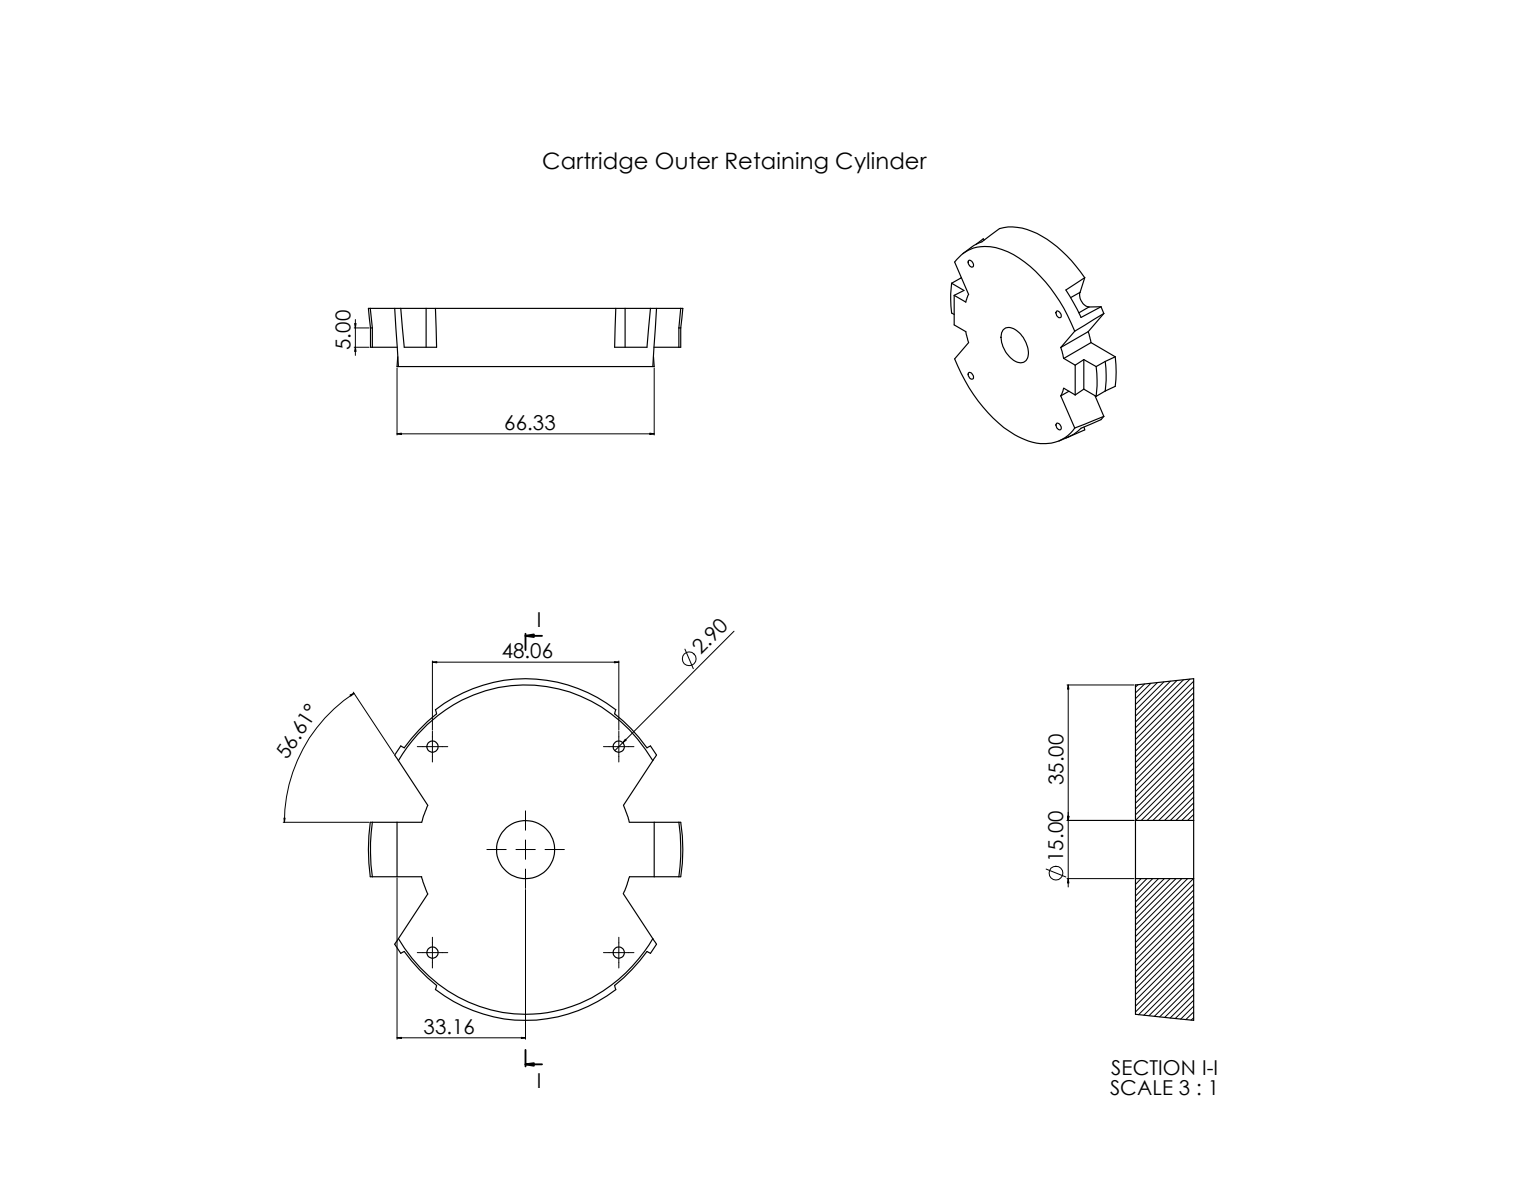
ISO-10303-21;
HEADER;
FILE_DESCRIPTION (('STEP AP214'),
    '1' );
FILE_NAME ('Cartridge Outer Retaining Cylinder.step',
    '2026-10-18T20:16:25',
    ( '' ),
    ( '' ),
    'SwSTEP 2.0',
    'SolidWorks 2025',
    '' );
FILE_SCHEMA (( 'AUTOMOTIVE_DESIGN' ));
ENDSEC;

DATA;
#17=CARTESIAN_POINT ( 'NONE',  ( -9.060903275275968838, 42.96476308719554993, -16.50000000000000000 ) ) ;
#22=EDGE_CURVE ( 'NONE', #25287, #29372, #18804, .T. ) ;
#32=CARTESIAN_POINT ( 'NONE',  ( -20.65888525914364493, -38.75220717792906555, -19.50000000000000355 ) ) ;
#41=CARTESIAN_POINT ( 'NONE',  ( 39.83602371821015709, 11.57901747687536265, -19.50000000000000355 ) ) ;
#46=CARTESIAN_POINT ( 'NONE',  ( -24.03057240117690441, -26.57182937991348481, 26.54355021145563143 ) ) ;
#74=AXIS2_PLACEMENT_3D ( 'NONE', #21270, #28002, #15999 ) ;
#78=DIRECTION ( 'NONE',  ( -1.000000000000000000, 0.000000000000000000, 0.000000000000000000 ) ) ;
#85=CARTESIAN_POINT ( 'NONE',  ( -37.98493438988125348, -11.12428508575252728, -1.500000000000000000 ) ) ;
#92=EDGE_CURVE ( 'NONE', #21118, #30725, #17328, .T. ) ;
#102=CARTESIAN_POINT ( 'NONE',  ( 22.58267429318970443, -26.57182937991349903, 26.54355021145563143 ) ) ;
#111=ORIENTED_EDGE ( 'NONE', *, *, #4642, .T. ) ;
#123=ORIENTED_EDGE ( 'NONE', *, *, #26128, .F. ) ;
#145=LINE ( 'NONE', #9510, #21267 ) ;
#162=AXIS2_PLACEMENT_3D ( 'NONE', #23397, #25742, #23542 ) ;
#169=CARTESIAN_POINT ( 'NONE',  ( 32.24119435725080507, -26.76047165977712794, -16.50000600000000262 ) ) ;
#175=CARTESIAN_POINT ( 'NONE',  ( -10.64374042650075403, -42.96126232887726815, -19.50000000000000355 ) ) ;
#176=CARTESIAN_POINT ( 'NONE',  ( 39.70095622563236049, 7.028748154183632302, -13.16666434799647689 ) ) ;
#184=CARTESIAN_POINT ( 'NONE',  ( -35.76344986165604212, -22.29344514668547461, -19.50000000000000355 ) ) ;
#187=EDGE_CURVE ( 'NONE', #14088, #4162, #7585, .T. ) ;
#226=CARTESIAN_POINT ( 'NONE',  ( 4.770489558936219510E-15, -42.50000000000000000, -1.500000000000000000 ) ) ;
#229=DIRECTION ( 'NONE',  ( -0.000000000000000000, -0.000000000000000000, -1.000000000000000000 ) ) ;
#231=CARTESIAN_POINT ( 'NONE',  ( 32.74775157611827581, 27.21557300921217859, -19.50000000000000355 ) ) ;
#253=CARTESIAN_POINT ( 'NONE',  ( 11.29353189506152511, 42.33618545487009754, -16.50000000000000355 ) ) ;
#258=PLANE ( 'NONE',  #5321 ) ;
#261=PLANE ( 'NONE',  #7575 ) ;
#285=CARTESIAN_POINT ( 'NONE',  ( 31.61046531718064045, -26.43913157134468861, -9.833326303308560057 ) ) ;
#301=CARTESIAN_POINT ( 'NONE',  ( 39.52380524535330153, 7.028748154198969367, -6.500000000000000888 ) ) ;
#313=AXIS2_PLACEMENT_3D ( 'NONE', #7814, #17164, #27009 ) ;
#326=VECTOR ( 'NONE', #28352, 1000.000000000000000 ) ;
#331=AXIS2_PLACEMENT_3D ( 'NONE', #19612, #5728, #15222 ) ;
#333=CARTESIAN_POINT ( 'NONE',  ( -39.00000000000000000, 5.563236990218665134, -1.500000000000000000 ) ) ;
#334=DIRECTION ( 'NONE',  ( 1.000000000000000000, 0.000000000000000000, 0.000000000000000000 ) ) ;
#335=ORIENTED_EDGE ( 'NONE', *, *, #27473, .T. ) ;
#342=CARTESIAN_POINT ( 'NONE',  ( -19.64114023396061981, 37.13592150528867109, -1.500000000000000000 ) ) ;
#347=CARTESIAN_POINT ( 'NONE',  ( 33.67904611720809527, -24.24635140547922418, -14.83330431372250935 ) ) ;
#349=AXIS2_PLACEMENT_3D ( 'NONE', #29658, #10628, #8296 ) ;
#401=CARTESIAN_POINT ( 'NONE',  ( -33.78553954455730235, -24.40792764007751359, -16.50000000000000000 ) ) ;
#407=LINE ( 'NONE', #9924, #2084 ) ;
#434=EDGE_LOOP ( 'NONE', ( #12928, #30003 ) ) ;
#443=DIRECTION ( 'NONE',  ( -0.000000000000000000, -0.000000000000000000, 1.000000000000000000 ) ) ;
#448=ORIENTED_EDGE ( 'NONE', *, *, #24131, .T. ) ;
#455=EDGE_CURVE ( 'NONE', #752, #3032, #6774, .T. ) ;
#471=DIRECTION ( 'NONE',  ( -0.8910248307962437275, 0.4539545692076742966, 0.000000000000000000 ) ) ;
#477=VERTEX_POINT ( 'NONE', #3410 ) ;
#484=LINE ( 'NONE', #7511, #24812 ) ;
#496=CARTESIAN_POINT ( 'NONE',  ( -10.64374042650306862, 42.96126232887723972, -19.50000000000000355 ) ) ;
#503=CARTESIAN_POINT ( 'NONE',  ( -5.105024945673440229, 42.22604126506271172, -1.500000000000000000 ) ) ;
#510=CARTESIAN_POINT ( 'NONE',  ( -33.78553954455730235, -24.40792764007751359, -16.50000000000000000 ) ) ;
#522=CARTESIAN_POINT ( 'NONE',  ( -24.03057240117690441, -26.57182937991348481, -6.499999999999999112 ) ) ;
#534=ORIENTED_EDGE ( 'NONE', *, *, #649, .F. ) ;
#544=VERTEX_POINT ( 'NONE', #30627 ) ;
#546=CARTESIAN_POINT ( 'NONE',  ( -33.57242512144540569, -24.08458161880429316, -13.16663720046962816 ) ) ;
#559=FACE_BOUND ( 'NONE', #17141, .T. ) ;
#571=CARTESIAN_POINT ( 'NONE',  ( 25.47847050916411504, 26.57182937991349903, -6.499999999999999112 ) ) ;
#601=ORIENTED_EDGE ( 'NONE', *, *, #19478, .T. ) ;
#626=ADVANCED_FACE ( 'NONE', ( #10658 ), #17680, .F. ) ;
#645=CARTESIAN_POINT ( 'NONE',  ( -26.80246859415415273, 7.028748154183637631, -1.499999999999999556 ) ) ;
#649=EDGE_CURVE ( 'NONE', #21864, #12141, #26737, .T. ) ;
#653=CARTESIAN_POINT ( 'NONE',  ( -39.00000000000000000, 5.563236990218665134, -1.500000000000000000 ) ) ;
#709=ORIENTED_EDGE ( 'NONE', *, *, #2670, .T. ) ;
#721=ADVANCED_FACE ( 'NONE', ( #3498 ), #3184, .T. ) ;
#730=PLANE ( 'NONE',  #331 ) ;
#732=CARTESIAN_POINT ( 'NONE',  ( 40.35867887216814864, 4.697862823546318012, -16.50000000000000000 ) ) ;
#752=VERTEX_POINT ( 'NONE', #835 ) ;
#762=CARTESIAN_POINT ( 'NONE',  ( -31.45274955327688460, -26.35877938677512233, -8.166661938620272565 ) ) ;
#769=ORIENTED_EDGE ( 'NONE', *, *, #21940, .F. ) ;
#792=CARTESIAN_POINT ( 'NONE',  ( 4.336808689942017736E-16, 42.50000000000000000, -1.500000000000000000 ) ) ;
#797=CARTESIAN_POINT ( 'NONE',  ( 0.000000000000000000, 0.000000000000000000, -1.500000000000000000 ) ) ;
#802=CARTESIAN_POINT ( 'NONE',  ( 10.11202017158399968, 41.14070756921128691, -1.500000000000000000 ) ) ;
#812=CARTESIAN_POINT ( 'NONE',  ( 32.82330813384209023, -22.94799032726822929, -1.500000000000000000 ) ) ;
#814=CARTESIAN_POINT ( 'NONE',  ( 32.51029041841470502, 26.37763988598561937, -16.50000000000000000 ) ) ;
#828=CARTESIAN_POINT ( 'NONE',  ( -20.71335220384823117, 27.86167394782616213, -16.50000600000000262 ) ) ;
#835=CARTESIAN_POINT ( 'NONE',  ( -33.16313691975489064, 7.028748154183637631, -1.500000000000000000 ) ) ;
#844=CARTESIAN_POINT ( 'NONE',  ( 5.105024945674004222, 42.22604126506330857, -1.500000000000000000 ) ) ;
#898=EDGE_LOOP ( 'NONE', ( #12196, #14932, #9204, #16861 ) ) ;
#911=CARTESIAN_POINT ( 'NONE',  ( 31.45274955338841494, -26.35877938683194088, -8.166661939779828572 ) ) ;
#924=AXIS2_PLACEMENT_3D ( 'NONE', #17670, #19692, #8017 ) ;
#981=DIRECTION ( 'NONE',  ( -0.8910248307962436165, -0.4539545692076747407, -0.000000000000000000 ) ) ;
#1013=CARTESIAN_POINT ( 'NONE',  ( -39.83602371821029919, -11.57901747687044924, -19.50000000000000355 ) ) ;
#1051=FACE_OUTER_BOUND ( 'NONE', #29406, .T. ) ;
#1052=EDGE_CURVE ( 'NONE', #4045, #16098, #4383, .T. ) ;
#1095=B_SPLINE_CURVE_WITH_KNOTS ( 'NONE', 3,
 ( #4359, #13883, #26037, #23676 ),
 .UNSPECIFIED., .F., .F.,
 ( 4, 4 ),
 ( 0.000000000000000000, 0.1536962897835600916 ),
 .UNSPECIFIED. ) ;
#1111=CARTESIAN_POINT ( 'NONE',  ( 29.15452456067735199, 29.11038375076175555, -6.500000000000000888 ) ) ;
#1115=CARTESIAN_POINT ( 'NONE',  ( -19.64114023396061981, 37.13592150528867109, -1.500000000000000000 ) ) ;
#1116=FACE_OUTER_BOUND ( 'NONE', #26170, .T. ) ;
#1153=EDGE_CURVE ( 'NONE', #11716, #4151, #9442, .T. ) ;
#1156=CARTESIAN_POINT ( 'NONE',  ( -35.76344986165608475, 22.29344514668535027, -19.50000000000000355 ) ) ;
#1162=CARTESIAN_POINT ( 'NONE',  ( 10.11202017158399968, 41.14070756921128691, -1.500000000000000000 ) ) ;
#1170=CARTESIAN_POINT ( 'NONE',  ( 5.374868878255610660, 44.10336124695606230, -19.50000000000000355 ) ) ;
#1181=DIRECTION ( 'NONE',  ( 0.000000000000000000, 0.000000000000000000, -1.000000000000000000 ) ) ;
#1199=EDGE_CURVE ( 'NONE', #24108, #2130, #15785, .T. ) ;
#1208=CARTESIAN_POINT ( 'NONE',  ( 25.19442432473618254, -35.44676296258426618, -19.50000000000000355 ) ) ;
#1246=ORIENTED_EDGE ( 'NONE', *, *, #13192, .F. ) ;
#1260=LINE ( 'NONE', #29338, #27317 ) ;
#1282=LINE ( 'NONE', #15460, #19231 ) ;
#1300=CARTESIAN_POINT ( 'NONE',  ( -24.98398214727286515, 23.12412086524405908, -16.50001200000000523 ) ) ;
#1302=CARTESIAN_POINT ( 'NONE',  ( -12.33859880789482233, 8.132258305203423632, -1.500000000000000000 ) ) ;
#1308=AXIS2_PLACEMENT_3D ( 'NONE', #17106, #19296, #2769 ) ;
#1310=CARTESIAN_POINT ( 'NONE',  ( -35.78163722268750746, -27.43648963448195133, -11.49999999999999645 ) ) ;
#1311=CARTESIAN_POINT ( 'NONE',  ( 35.76344986163714168, -22.29344514668044752, -19.50000000000000355 ) ) ;
#1317=CARTESIAN_POINT ( 'NONE',  ( -5.105024945675580739, -42.22604126506273303, -1.500000000000000000 ) ) ;
#1322=FACE_OUTER_BOUND ( 'NONE', #29141, .T. ) ;
#1332=CARTESIAN_POINT ( 'NONE',  ( 26.80246859415415273, -7.028748154183637631, -16.50000000000000000 ) ) ;
#1335=PLANE ( 'NONE',  #29203 ) ;
#1357=CARTESIAN_POINT ( 'NONE',  ( -40.89187623478217404, 5.790488632116478129, -19.50000000000000355 ) ) ;
#1362=CARTESIAN_POINT ( 'NONE',  ( 23.27838111857050407, -36.10018641471199174, -16.50000599999999906 ) ) ;
#1378=CARTESIAN_POINT ( 'NONE',  ( 24.03057240117691862, -26.57182937991349903, -6.500000000000000888 ) ) ;
#1393=ORIENTED_EDGE ( 'NONE', *, *, #9979, .F. ) ;
#1401=ORIENTED_EDGE ( 'NONE', *, *, #20994, .F. ) ;
#1408=CIRCLE ( 'NONE', #17835, 27.70876437800068359 ) ;
#1421=ADVANCED_FACE ( 'NONE', ( #4031 ), #18074, .F. ) ;
#1434=CARTESIAN_POINT ( 'NONE',  ( -26.80246859415415273, 7.028748154183637631, -16.50000000000000000 ) ) ;
#1466=CARTESIAN_POINT ( 'NONE',  ( -22.85987860430571317, -23.19171692911513460, -16.50001200000000168 ) ) ;
#1475=LINE ( 'NONE', #15646, #18551 ) ;
#1477=CARTESIAN_POINT ( 'NONE',  ( 2.687479362164894248, -44.39187623478217404, -19.50000000000000355 ) ) ;
#1482=CARTESIAN_POINT ( 'NONE',  ( -39.83602371821034183, 11.57901747687032490, -19.50000000000000355 ) ) ;
#1484=CARTESIAN_POINT ( 'NONE',  ( 24.03057240117691862, 26.57182937991349903, -6.499999999999999112 ) ) ;
#1488=CARTESIAN_POINT ( 'NONE',  ( 39.00000000000000000, -5.563236990218592304, -1.500000000000000000 ) ) ;
#1512=DIRECTION ( 'NONE',  ( 0.5503133621338236470, -0.8349582046168341209, -0.000000000000000000 ) ) ;
#1516=CARTESIAN_POINT ( 'NONE',  ( -32.74775157610409337, 27.21557300919391054, -19.50000000000000355 ) ) ;
#1569=EDGE_LOOP ( 'NONE', ( #15158, #10530, #11871, #10690 ) ) ;
#1574=B_SPLINE_CURVE_WITH_KNOTS ( 'NONE', 3,
 ( #9873, #15005, #12688, #10176, #510 ),
 .UNSPECIFIED., .F., .F.,
 ( 4, 1, 4 ),
 ( 0.1429309129599393158, 0.1481973127024909243, 0.1534637124450425050 ),
 .UNSPECIFIED. ) ;
#1602=AXIS2_PLACEMENT_3D ( 'NONE', #1378, #19360, #7512 ) ;
#1605=CARTESIAN_POINT ( 'NONE',  ( 39.87350638640253919, -4.706224724400463799, -6.500000000000000888 ) ) ;
#1621=ORIENTED_EDGE ( 'NONE', *, *, #4317, .F. ) ;
#1629=CARTESIAN_POINT ( 'NONE',  ( -19.64114023396061981, 37.13592150528867109, -1.500000000000000000 ) ) ;
#1630=CARTESIAN_POINT ( 'NONE',  ( -22.94541271838176044, 35.03073867844246081, -6.500000000000000888 ) ) ;
#1639=CARTESIAN_POINT ( 'NONE',  ( -5.374868878256215510, -44.10336124695545124, -19.50000000000000355 ) ) ;
#1654=CARTESIAN_POINT ( 'NONE',  ( 24.73258466867350336, -33.64422401625958514, -6.500000000000000888 ) ) ;
#1655=CARTESIAN_POINT ( 'NONE',  ( 35.78163722268750746, 27.43648963448195133, -11.49999999999999645 ) ) ;
#1667=CARTESIAN_POINT ( 'NONE',  ( 24.03057240117691862, 26.57182937991349903, -6.500000000000000888 ) ) ;
#1750=ADVANCED_FACE ( 'NONE', ( #21628, #14614 ), #24117, .T. ) ;
#1754=CARTESIAN_POINT ( 'NONE',  ( -25.64627119138473432, -23.40052582045089480, -16.50000600000000262 ) ) ;
#1756=ADVANCED_FACE ( 'NONE', ( #10234 ), #12279, .F. ) ;
#1757=CARTESIAN_POINT ( 'NONE',  ( 24.03057240117690441, -26.57182937991349903, 26.54355021145563143 ) ) ;
#1763=CARTESIAN_POINT ( 'NONE',  ( 0.000000000000000000, 44.39187623478217404, -19.50000000000000355 ) ) ;
#1781=CARTESIAN_POINT ( 'NONE',  ( -2.687479363073305372, 44.39187623477332068, -19.50000000000000355 ) ) ;
#1812=CARTESIAN_POINT ( 'NONE',  ( 33.67904611717059993, 24.24635140542181233, -14.83330431306680453 ) ) ;
#1847=CIRCLE ( 'NONE', #17271, 27.70876437800068359 ) ;
#1863=VERTEX_POINT ( 'NONE', #23003 ) ;
#1864=CARTESIAN_POINT ( 'NONE',  ( -24.73258466867759608, 33.64422401626517001, -6.500000000000000888 ) ) ;
#1869=LINE ( 'NONE', #6846, #8646 ) ;
#1896=EDGE_LOOP ( 'NONE', ( #27103, #9157, #6706, #24049 ) ) ;
#1902=CARTESIAN_POINT ( 'NONE',  ( -20.29038667444665833, 38.16990472509154841, -16.50000000000000000 ) ) ;
#1907=CARTESIAN_POINT ( 'NONE',  ( -24.98398214727285804, -23.12412086524405908, -16.50001200000000523 ) ) ;
#1908=CARTESIAN_POINT ( 'NONE',  ( -25.64627119138473788, 23.40052582045089480, -16.50000000000000000 ) ) ;
#1912=ORIENTED_EDGE ( 'NONE', *, *, #28902, .T. ) ;
#1932=CARTESIAN_POINT ( 'NONE',  ( -23.96732207938974213, -33.98584080153308662, -1.500000000000000000 ) ) ;
#1958=LINE ( 'NONE', #18960, #28468 ) ;
#1961=DIRECTION ( 'NONE',  ( 0.000000000000000000, 1.000000000000000000, -0.000000000000000000 ) ) ;
#1964=CARTESIAN_POINT ( 'NONE',  ( 12.56641067637628240, -40.32935944494942504, -1.500000000000000000 ) ) ;
#1966=CARTESIAN_POINT ( 'NONE',  ( -26.80246859415415273, -7.028748154183645624, -1.499999999999999556 ) ) ;
#1970=CIRCLE ( 'NONE', #4441, 1.447898107987198646 ) ;
#1976=EDGE_CURVE ( 'NONE', #12213, #16156, #16385, .T. ) ;
#1989=CARTESIAN_POINT ( 'NONE',  ( 23.06931171825916493, -36.25841434086032677, -16.50000000000000000 ) ) ;
#2009=B_SPLINE_CURVE_WITH_KNOTS ( 'NONE', 3,
 ( #16990, #26512, #16530, #11702, #7021, #23395, #2033, #28545, #21360, #11557 ),
 .UNSPECIFIED., .F., .F.,
 ( 4, 2, 2, 2, 4 ),
 ( 0.08772604163077325767, 0.09629186329443806258, 0.1119390432090576204, 0.1197626331663674271, 0.1275862231236772337 ),
 .UNSPECIFIED. ) ;
#2012=CARTESIAN_POINT ( 'NONE',  ( -24.03057240117691862, 26.57182937991348481, 26.54355021145563143 ) ) ;
#2016=ORIENTED_EDGE ( 'NONE', *, *, #30517, .T. ) ;
#2033=CARTESIAN_POINT ( 'NONE',  ( -10.11202017158466759, 41.14070756921185534, -1.500000000000009992 ) ) ;
#2047=CARTESIAN_POINT ( 'NONE',  ( -19.05926965620446722, 38.91648619949726395, -16.49999999999999289 ) ) ;
#2050=CARTESIAN_POINT ( 'NONE',  ( -39.52380524535562500, 7.028748154183637631, -11.49999999999999645 ) ) ;
#2075=CARTESIAN_POINT ( 'NONE',  ( -34.07766914599908148, -21.40380666528021081, -1.500000000000000000 ) ) ;
#2076=LINE ( 'NONE', #25500, #21890 ) ;
#2084=VECTOR ( 'NONE', #19436, 1000.000000000000000 ) ;
#2093=PRODUCT_DEFINITION ( 'UNKNOWN', '', #6419, #16060 ) ;
#2099=LINE ( 'NONE', #11622, #24469 ) ;
#2109=CARTESIAN_POINT ( 'NONE',  ( -25.19442432475839055, 35.44676296258369064, -19.50000000000000355 ) ) ;
#2127=AXIS2_PLACEMENT_3D ( 'NONE', #16002, #25522, #22698 ) ;
#2130=VERTEX_POINT ( 'NONE', #14428 ) ;
#2131=CARTESIAN_POINT ( 'NONE',  ( -32.82330813384395185, 22.94799032727105370, -1.500000000000000000 ) ) ;
#2135=CARTESIAN_POINT ( 'NONE',  ( 5.229169525036386545, -43.72378943593913192, -16.49999999999999289 ) ) ;
#2161=CARTESIAN_POINT ( 'NONE',  ( 0.000000000000000000, 0.000000000000000000, -16.50000000000000000 ) ) ;
#2195=CARTESIAN_POINT ( 'NONE',  ( 40.05104235265675783, -2.353288714521556191, -6.500000000000000888 ) ) ;
#2214=CARTESIAN_POINT ( 'NONE',  ( 2.552544031601107211, 42.49999999998228617, -1.500000000000000000 ) ) ;
#2215=FACE_OUTER_BOUND ( 'NONE', #8737, .T. ) ;
#2221=CARTESIAN_POINT ( 'NONE',  ( 35.76344986165623396, 22.29344514668041199, -19.50000000000000355 ) ) ;
#2227=ORIENTED_EDGE ( 'NONE', *, *, #29644, .F. ) ;
#2231=VERTEX_POINT ( 'NONE', #10865 ) ;
#2242=DIRECTION ( 'NONE',  ( 1.000000000000000000, -1.559722691008415723E-11, 0.000000000000000000 ) ) ;
#2254=CARTESIAN_POINT ( 'NONE',  ( 32.82330813384209023, -22.94799032726822929, -1.500000000000000000 ) ) ;
#2258=CARTESIAN_POINT ( 'NONE',  ( 5.105024945674004222, 42.22604126506330857, -1.500000000000000000 ) ) ;
#2259=DIRECTION ( 'NONE',  ( -0.000000000000000000, -0.000000000000000000, -1.000000000000000000 ) ) ;
#2261=VERTEX_POINT ( 'NONE', #13366 ) ;
#2270=CARTESIAN_POINT ( 'NONE',  ( -21.58118279630250314, -37.32782027973600947, -16.50000000000000000 ) ) ;
#2292=VERTEX_POINT ( 'NONE', #26986 ) ;
#2297=( NAMED_UNIT ( * ) PLANE_ANGLE_UNIT ( ) SI_UNIT ( $, .RADIAN. ) );
#2298=VERTEX_POINT ( 'NONE', #18040 ) ;
#2305=CARTESIAN_POINT ( 'NONE',  ( 32.24119409414369386, 26.76047229433004659, -16.50000600000000262 ) ) ;
#2332=CARTESIAN_POINT ( 'NONE',  ( 40.05104235265675783, -2.353288714521559744, -11.49999999999999645 ) ) ;
#2355=CARTESIAN_POINT ( 'NONE',  ( -19.85060193104290960, 38.44128451546529845, -16.49999999999999645 ) ) ;
#2366=FACE_OUTER_BOUND ( 'NONE', #5694, .T. ) ;
#2371=CARTESIAN_POINT ( 'NONE',  ( 23.96732207937828463, 33.98584080152456011, -1.500000000000000000 ) ) ;
#2382=CARTESIAN_POINT ( 'NONE',  ( 13.22505861668094340, 42.10773672057246841, -19.50000000000000355 ) ) ;
#2393=CARTESIAN_POINT ( 'NONE',  ( -5.105024945675580739, -42.22604126506273303, -1.500000000000000000 ) ) ;
#2404=VECTOR ( 'NONE', #10692, 1000.000000000000114 ) ;
#2405=LINE ( 'NONE', #17052, #29792 ) ;
#2425=VERTEX_POINT ( 'NONE', #7566 ) ;
#2428=CARTESIAN_POINT ( 'NONE',  ( -19.64114023396299302, -37.13592150529018454, -1.500000000000000000 ) ) ;
#2440=CARTESIAN_POINT ( 'NONE',  ( -33.35889462893121049, -23.76060431981724363, -9.833271596736169684 ) ) ;
#2442=LINE ( 'NONE', #11963, #7867 ) ;
#2478=CARTESIAN_POINT ( 'NONE',  ( 25.23756106473024019, 11.43858098102958287, -11.49999999999999645 ) ) ;
#2482=DIRECTION ( 'NONE',  ( -0.000000000000000000, -0.000000000000000000, -1.000000000000000000 ) ) ;
#2496=CARTESIAN_POINT ( 'NONE',  ( -40.05520443301966083, -7.028746486913004077, -16.50000000000000000 ) ) ;
#2497=CARTESIAN_POINT ( 'NONE',  ( 20.62927206985200712, -25.36120318786823802, -16.50001200000000523 ) ) ;
#2503=ADVANCED_FACE ( 'NONE', ( #10514 ), #6662, .T. ) ;
#2527=CARTESIAN_POINT ( 'NONE',  ( -24.73258466867722660, -33.64422401626472237, -6.500000000000000888 ) ) ;
#2532=CARTESIAN_POINT ( 'NONE',  ( -2.687479363073305372, 44.39187623477332068, -19.50000000000000355 ) ) ;
#2541=CARTESIAN_POINT ( 'NONE',  ( -39.00000000000000000, -5.563236990218529243, -1.500000000000000000 ) ) ;
#2553=CARTESIAN_POINT ( 'NONE',  ( -24.03057240117691862, -26.57182937991349903, -6.500000000000000888 ) ) ;
#2557=EDGE_LOOP ( 'NONE', ( #20705, #9961, #8594, #30062 ) ) ;
#2580=ORIENTED_EDGE ( 'NONE', *, *, #22101, .T. ) ;
#2594=CARTESIAN_POINT ( 'NONE',  ( -22.43745300381736030, -36.72714324444464040, -16.50000000000000000 ) ) ;
#2599=CARTESIAN_POINT ( 'NONE',  ( 16.14703582738955490, 40.45263314063372206, -16.50000000000000711 ) ) ;
#2645=ORIENTED_EDGE ( 'NONE', *, *, #23070, .F. ) ;
#2654=MANIFOLD_SOLID_BREP ( 'Cut-Extrude13', #3869 ) ;
#2658=EDGE_CURVE ( 'NONE', #16156, #16328, #1282, .T. ) ;
#2670=EDGE_CURVE ( 'NONE', #477, #1863, #17345, .T. ) ;
#2679=CARTESIAN_POINT ( 'NONE',  ( -37.98493438988125348, -11.12428508575252728, -1.500000000000000000 ) ) ;
#2690=CARTESIAN_POINT ( 'NONE',  ( 34.07766914600081520, 21.40380666527109810, -1.500000000000000000 ) ) ;
#2698=CYLINDRICAL_SURFACE ( 'NONE', #27387, 3.559164065751841743 ) ;
#2699=ORIENTED_EDGE ( 'NONE', *, *, #23180, .F. ) ;
#2721=CARTESIAN_POINT ( 'NONE',  ( 24.03057240117691862, 26.57182937991349903, -6.500000000000000888 ) ) ;
#2752=ORIENTED_EDGE ( 'NONE', *, *, #25397, .F. ) ;
#2756=CARTESIAN_POINT ( 'NONE',  ( 18.46022885586396356, 39.25482954210340125, -16.49999999999999645 ) ) ;
#2766=DIRECTION ( 'NONE',  ( -0.000000000000000000, -0.000000000000000000, -1.000000000000000000 ) ) ;
#2769=DIRECTION ( 'NONE',  ( -1.000000000000000000, 0.000000000000000000, 0.000000000000000000 ) ) ;
#2815=CARTESIAN_POINT ( 'NONE',  ( 5.204170427930421283E-15, -44.07656352898514740, -16.50000000000000000 ) ) ;
#2823=AXIS2_PLACEMENT_3D ( 'NONE', #19081, #25384, #23019 ) ;
#2824=FACE_OUTER_BOUND ( 'NONE', #13856, .T. ) ;
#2827=CARTESIAN_POINT ( 'NONE',  ( -24.03057240117691862, 26.57182937991348481, -1.500000000000001332 ) ) ;
#2836=CARTESIAN_POINT ( 'NONE',  ( -13.22505861668184046, -42.10773672057003125, -19.50000000000000355 ) ) ;
#2837=CARTESIAN_POINT ( 'NONE',  ( 40.05520497557499482, 7.028746409576331011, -16.50000000000000000 ) ) ;
#2844=CARTESIAN_POINT ( 'NONE',  ( -39.83602371821034183, 11.57901747687032490, -19.50000000000000355 ) ) ;
#2867=CARTESIAN_POINT ( 'NONE',  ( -23.20738078402527549, 23.09073189384302793, -16.50001200000000168 ) ) ;
#2870=CARTESIAN_POINT ( 'NONE',  ( 11.46038621610576236, -42.28394141292588415, -16.50000000000000000 ) ) ;
#2891=EDGE_CURVE ( 'NONE', #25287, #18178, #3562, .T. ) ;
#2900=VECTOR ( 'NONE', #14038, 1000.000000000000114 ) ;
#2902=ORIENTED_EDGE ( 'NONE', *, *, #8502, .F. ) ;
#2912=EDGE_CURVE ( 'NONE', #30328, #18557, #9016, .T. ) ;
#2915=ORIENTED_EDGE ( 'NONE', *, *, #25460, .F. ) ;
#2917=FACE_BOUND ( 'NONE', #16843, .T. ) ;
#2922=DIRECTION ( 'NONE',  ( -1.000000000000000000, 0.000000000000000000, -0.000000000000000000 ) ) ;
#2936=DIRECTION ( 'NONE',  ( -0.000000000000000000, -0.000000000000000000, 1.000000000000000000 ) ) ;
#2995=CARTESIAN_POINT ( 'NONE',  ( 0.000000000000000000, 0.000000000000000000, -1.500000000000001332 ) ) ;
#3001=ORIENTED_EDGE ( 'NONE', *, *, #27898, .T. ) ;
#3006=CARTESIAN_POINT ( 'NONE',  ( 37.98493438989863336, -11.12428508576153341, -1.500000000000000000 ) ) ;
#3007=DIRECTION ( 'NONE',  ( 1.000000000000000000, 0.000000000000000000, 0.000000000000000000 ) ) ;
#3012=ORIENTED_EDGE ( 'NONE', *, *, #18180, .F. ) ;
#3022=CARTESIAN_POINT ( 'NONE',  ( -39.52380524535562500, 7.028748154183637631, -1.499999999999999556 ) ) ;
#3032=VERTEX_POINT ( 'NONE', #16643 ) ;
#3060=CARTESIAN_POINT ( 'NONE',  ( 5.184529477212510784, 43.72990366966700293, -16.50000000000000000 ) ) ;
#3075=ADVANCED_FACE ( 'NONE', ( #21464, #14750, #10079, #559, #2917, #18990 ), #258, .F. ) ;
#3079=DIRECTION ( 'NONE',  ( -1.000000000000000000, 0.000000000000000000, 0.000000000000000000 ) ) ;
#3108=LINE ( 'NONE', #24769, #14010 ) ;
#3125=ORIENTED_EDGE ( 'NONE', *, *, #26838, .F. ) ;
#3129=ORIENTED_EDGE ( 'NONE', *, *, #29186, .T. ) ;
#3148=CARTESIAN_POINT ( 'NONE',  ( -23.96732207939035675, 33.98584080153585774, -1.500000000000000000 ) ) ;
#3156=CARTESIAN_POINT ( 'NONE',  ( -13.22505861668333083, 42.10773672057167261, -19.50000000000000355 ) ) ;
#3165=CARTESIAN_POINT ( 'NONE',  ( 33.25198513809822742, -23.59839681648444554, -8.166573414591441704 ) ) ;
#3176=CARTESIAN_POINT ( 'NONE',  ( 39.52380524535562500, 7.028748154183637631, -6.500000000000000888 ) ) ;
#3184=PLANE ( 'NONE',  #25082 ) ;
#3191=CARTESIAN_POINT ( 'NONE',  ( 2.552544031601107211, 42.49999999998228617, -1.500000000000000000 ) ) ;
#3217=CARTESIAN_POINT ( 'NONE',  ( -26.80246859415415273, 7.028748154183637631, -1.499999999999999556 ) ) ;
#3270=CARTESIAN_POINT ( 'NONE',  ( -20.71335220384823117, 27.86167394782616213, -16.50000600000000262 ) ) ;
#3296=VERTEX_POINT ( 'NONE', #21107 ) ;
#3328=CARTESIAN_POINT ( 'NONE',  ( -22.58267429318971864, 26.57182937991348481, -1.500000000000001332 ) ) ;
#3340=CARTESIAN_POINT ( 'NONE',  ( 31.18700685317242716, 26.11823559933198879, -1.500000000000000000 ) ) ;
#3346=CARTESIAN_POINT ( 'NONE',  ( -31.18700685316100163, -26.11823559932341610, -1.500000000000000000 ) ) ;
#3370=VECTOR ( 'NONE', #14525, 1000.000000000000114 ) ;
#3380=ORIENTED_EDGE ( 'NONE', *, *, #1052, .F. ) ;
#3394=ORIENTED_EDGE ( 'NONE', *, *, #19459, .F. ) ;
#3398=CARTESIAN_POINT ( 'NONE',  ( 40.56744461766400178, 1.008925180279410139, -16.50000000000000000 ) ) ;
#3404=EDGE_LOOP ( 'NONE', ( #25073, #1401, #3581, #18257, #26796, #15185, #9678, #9859, #11224, #26072, #16671, #534, #335, #23589, #5816, #30130, #28609, #20043, #22288, #9616, #21858, #17373, #5302, #7145, #17610, #15610, #17048, #1393, #16611, #14155, #14862, #18230, #16761, #17005, #27766, #9497 ) ) ;
#3410=CARTESIAN_POINT ( 'NONE',  ( -25.64627119138473788, 23.40052582045089480, -16.50000000000000000 ) ) ;
#3447=CARTESIAN_POINT ( 'NONE',  ( -26.80246859415415273, -7.028748154183637631, -1.499999999999999556 ) ) ;
#3498=FACE_OUTER_BOUND ( 'NONE', #18843, .T. ) ;
#3510=ORIENTED_EDGE ( 'NONE', *, *, #19853, .F. ) ;
#3512=CARTESIAN_POINT ( 'NONE',  ( 5.374868878254059013, -44.10336124695543703, -19.50000000000000355 ) ) ;
#3517=AXIS2_PLACEMENT_3D ( 'NONE', #29672, #17356, #13147 ) ;
#3519=CARTESIAN_POINT ( 'NONE',  ( -35.76344986165604212, -22.29344514668547461, -19.50000000000000355 ) ) ;
#3544=CARTESIAN_POINT ( 'NONE',  ( -35.76344986165604212, -22.29344514668547461, -19.50000000000000355 ) ) ;
#3562=LINE ( 'NONE', #7945, #13243 ) ;
#3571=DIRECTION ( 'NONE',  ( -1.000000000000000000, 0.000000000000000000, 0.000000000000000000 ) ) ;
#3580=CARTESIAN_POINT ( 'NONE',  ( -33.16313691975489064, -7.028748154183637631, -1.500000000000000000 ) ) ;
#3581=ORIENTED_EDGE ( 'NONE', *, *, #15915, .F. ) ;
#3604=CARTESIAN_POINT ( 'NONE',  ( 22.94541271837968566, 35.03073867843525591, -6.499999999999999112 ) ) ;
#3637=CARTESIAN_POINT ( 'NONE',  ( -23.22298177193101765, -35.92225147532004570, -14.83329744750909995 ) ) ;
#3659=CARTESIAN_POINT ( 'NONE',  ( 19.64114023396890829, 37.13592150528549496, -1.500000000000000000 ) ) ;
#3660=ADVANCED_FACE ( 'NONE', ( #20244 ), #29771, .T. ) ;
#3662=B_SPLINE_CURVE_WITH_KNOTS ( 'NONE', 3,
 ( #11603, #26682, #7661, #24012, #21523, #19358, #5312, #14520, #13945, #9842 ),
 .UNSPECIFIED., .F., .F.,
 ( 4, 3, 3, 4 ),
 ( -0.005033671592849668641, 0.000000000000000000, 0.005033946531780089662, 0.01006789358107974472 ),
 .UNSPECIFIED. ) ;
#3666=CARTESIAN_POINT ( 'NONE',  ( 12.56641067637329812, 40.32935944495179115, -1.500000000000000000 ) ) ;
#3709=DIRECTION ( 'NONE',  ( -1.000000000000000000, 0.000000000000000000, 0.000000000000000000 ) ) ;
#3721=EDGE_LOOP ( 'NONE', ( #8377, #22423, #28746, #15898 ) ) ;
#3734=PLANE ( 'NONE',  #12264 ) ;
#3753=VERTEX_POINT ( 'NONE', #30223 ) ;
#3795=CARTESIAN_POINT ( 'NONE',  ( -24.03057240117690441, -26.57182937991348481, 26.54355021145563143 ) ) ;
#3797=CARTESIAN_POINT ( 'NONE',  ( -20.71335220384823117, -27.86167394782616213, -16.50000000000000000 ) ) ;
#3806=CARTESIAN_POINT ( 'NONE',  ( -2.687479363073305372, 44.39187623477332068, -19.50000000000000355 ) ) ;
#3811=CARTESIAN_POINT ( 'NONE',  ( 23.96732207937828463, 33.98584080152456011, -1.500000000000000000 ) ) ;
#3817=CARTESIAN_POINT ( 'NONE',  ( 31.18700685317242716, 26.11823559933198879, -1.500000000000000000 ) ) ;
#3829=CARTESIAN_POINT ( 'NONE',  ( 1.734723475976807094E-15, -44.07656352898514740, -6.500000000000000888 ) ) ;
#3859=ORIENTED_EDGE ( 'NONE', *, *, #19661, .T. ) ;
#3861=VECTOR ( 'NONE', #12040, 1000.000000000000000 ) ;
#3869=CLOSED_SHELL ( 'NONE', ( #28448, #2503, #13583, #1756, #8857, #10128, #14330, #27072, #18523, #3075, #9353, #28639, #6406, #4777, #6909, #16272, #15303, #4583, #21564, #15221, #27786, #24242, #626, #1750, #15368, #25391, #20831, #21794, #15982, #23364, #9380, #8644, #8818, #20413, #8615, #9779, #23667, #27306, #5769, #29435, #25776, #12783, #18322, #8982, #7354, #30362, #5241, #3660, #17604, #1421, #24429, #721, #17780, #23893 ) ) ;
#3937=B_SPLINE_SURFACE_WITH_KNOTS ( 'NONE', 3, 1, ( 
 ( #28544, #28395 ),
 ( #30568, #23998 ),
 ( #19177, #2332 ),
 ( #18720, #4678 ),
 ( #28699, #14500 ),
 ( #301, #4827 ) ),
 .UNSPECIFIED., .F., .F., .F.,
 ( 4, 2, 4 ),
 ( 2, 2 ),
 ( 1.408367944307646891, 1.570796326794821507, 1.733224709277728426 ),
 ( 0.000000000000000000, 1.000000000000000000 ),
 .UNSPECIFIED. ) ;
#3940=AXIS2_PLACEMENT_3D ( 'NONE', #5168, #28727, #21687 ) ;
#3952=AXIS2_PLACEMENT_3D ( 'NONE', #11741, #30768, #25935 ) ;
#3969=CARTESIAN_POINT ( 'NONE',  ( 12.56641067637628240, -40.32935944494942504, -1.500000000000000000 ) ) ;
#3973=CARTESIAN_POINT ( 'NONE',  ( -32.74775157610409337, 27.21557300919391054, -19.50000000000000355 ) ) ;
#3979=CARTESIAN_POINT ( 'NONE',  ( 2.687479362164894248, -44.39187623478217404, -19.50000000000000355 ) ) ;
#4002=CARTESIAN_POINT ( 'NONE',  ( -40.05520443301966083, -7.028746486913004077, -16.50000000000000000 ) ) ;
#4025=CARTESIAN_POINT ( 'NONE',  ( 25.47847050916410439, -26.57182937991349903, 26.54355021145563143 ) ) ;
#4031=FACE_OUTER_BOUND ( 'NONE', #21646, .T. ) ;
#4035=ORIENTED_EDGE ( 'NONE', *, *, #10269, .T. ) ;
#4045=VERTEX_POINT ( 'NONE', #29895 ) ;
#4058=EDGE_CURVE ( 'NONE', #6837, #752, #27084, .T. ) ;
#4065=CARTESIAN_POINT ( 'NONE',  ( 31.29501345866090389, 26.27841684422296353, -6.500000000000000888 ) ) ;
#4079=LINE ( 'NONE', #13609, #19373 ) ;
#4084=EDGE_CURVE ( 'NONE', #15207, #7019, #19784, .T. ) ;
#4091=EDGE_LOOP ( 'NONE', ( #13530, #26791, #12899, #4967 ) ) ;
#4096=FACE_OUTER_BOUND ( 'NONE', #11719, .T. ) ;
#4111=CARTESIAN_POINT ( 'NONE',  ( -12.56641067637617759, -40.32935944494947478, -1.500000000000000000 ) ) ;
#4122=CARTESIAN_POINT ( 'NONE',  ( 12.33859880789485253, 8.132258305203430737, -16.50000000000000000 ) ) ;
#4124=CARTESIAN_POINT ( 'NONE',  ( -20.65888525914099105, 38.75220717792564784, -19.50000000000000355 ) ) ;
#4151=VERTEX_POINT ( 'NONE', #6485 ) ;
#4159=CARTESIAN_POINT ( 'NONE',  ( 26.80246859415415273, -7.028748154183637631, -6.500000000000000888 ) ) ;
#4162=VERTEX_POINT ( 'NONE', #18799 ) ;
#4169=CARTESIAN_POINT ( 'NONE',  ( 8.828055718019477638, -43.02192272134110596, -16.50000000000000000 ) ) ;
#4182=VERTEX_POINT ( 'NONE', #4453 ) ;
#4185=EDGE_CURVE ( 'NONE', #15872, #6674, #25382, .T. ) ;
#4208=ORIENTED_EDGE ( 'NONE', *, *, #6336, .T. ) ;
#4218=EDGE_CURVE ( 'NONE', #14001, #13970, #18775, .T. ) ;
#4230=ORIENTED_EDGE ( 'NONE', *, *, #2891, .T. ) ;
#4235=CARTESIAN_POINT ( 'NONE',  ( -20.94685371601454094, 37.75489722317177410, -16.49999999999998934 ) ) ;
#4242=DIRECTION ( 'NONE',  ( -0.000000000000000000, -0.000000000000000000, -1.000000000000000000 ) ) ;
#4250=ORIENTED_EDGE ( 'NONE', *, *, #17204, .F. ) ;
#4254=CARTESIAN_POINT ( 'NONE',  ( -2.552544031601109875, 42.50000000001772094, -1.500000000000000000 ) ) ;
#4264=VERTEX_POINT ( 'NONE', #29080 ) ;
#4269=ORIENTED_EDGE ( 'NONE', *, *, #6714, .T. ) ;
#4279=CARTESIAN_POINT ( 'NONE',  ( -20.71335220384823117, 27.86167394782616213, -16.50000000000000000 ) ) ;
#4296=CARTESIAN_POINT ( 'NONE',  ( -2.687479363073305372, 44.39187623477332068, -19.50000000000000355 ) ) ;
#4298=ORIENTED_EDGE ( 'NONE', *, *, #24131, .F. ) ;
#4307=CARTESIAN_POINT ( 'NONE',  ( -18.92920200386403451, -38.99007567941009711, -16.50000000000000000 ) ) ;
#4311=B_SPLINE_CURVE_WITH_KNOTS ( 'NONE', 3,
 ( #10305, #19822, #5118, #26332, #28979, #5270, #2305 ),
 .UNSPECIFIED., .F., .F.,
 ( 4, 3, 4 ),
 ( 0.000000000000000000, 0.005028111721475434122, 0.01005622344647096392 ),
 .UNSPECIFIED. ) ;
#4317=EDGE_CURVE ( 'NONE', #16098, #16473, #6136, .T. ) ;
#4325=VECTOR ( 'NONE', #2242, 1000.000000000000000 ) ;
#4332=CIRCLE ( 'NONE', #24257, 1.447898107987198646 ) ;
#4337=( NAMED_UNIT ( * ) SI_UNIT ( $, .STERADIAN. ) SOLID_ANGLE_UNIT ( ) );
#4345=LINE ( 'NONE', #11535, #19465 ) ;
#4350=AXIS2_PLACEMENT_3D ( 'NONE', #13291, #27633, #18117 ) ;
#4359=CARTESIAN_POINT ( 'NONE',  ( 20.71335220384823117, -27.86167394782616213, -16.50000600000000262 ) ) ;
#4369=EDGE_LOOP ( 'NONE', ( #25058, #111, #24453, #3394 ) ) ;
#4378=LINE ( 'NONE', #20906, #7453 ) ;
#4383=CIRCLE ( 'NONE', #21814, 7.500000000000000000 ) ;
#4385=CARTESIAN_POINT ( 'NONE',  ( 39.52380524533145945, -7.028748154382047808, -6.500000000000000888 ) ) ;
#4408=CARTESIAN_POINT ( 'NONE',  ( 13.22505861668094340, 42.10773672057246841, -19.50000000000000355 ) ) ;
#4414=CARTESIAN_POINT ( 'NONE',  ( -10.11202017158235833, -41.14070756921188377, -1.500000000000000000 ) ) ;
#4441=AXIS2_PLACEMENT_3D ( 'NONE', #15620, #20461, #29981 ) ;
#4443=ORIENTED_EDGE ( 'NONE', *, *, #19075, .F. ) ;
#4453=CARTESIAN_POINT ( 'NONE',  ( 25.47847050916411504, 26.57182937991349903, -1.500000000000001332 ) ) ;
#4459=PLANE ( 'NONE',  #20543 ) ;
#4463=CARTESIAN_POINT ( 'NONE',  ( 39.00000000000000000, -5.563236990218592304, -1.500000000000000000 ) ) ;
#4469=B_SPLINE_CURVE_WITH_KNOTS ( 'NONE', 1,
 ( #9085, #28113 ),
 .UNSPECIFIED., .F., .F.,
 ( 2, 2 ),
 ( 0.1666666666666667962, 1.000000000000000000 ),
 .UNSPECIFIED. ) ;
#4476=CARTESIAN_POINT ( 'NONE',  ( 24.03057240117690441, -26.57182937991349903, -6.499999999999999112 ) ) ;
#4477=CARTESIAN_POINT ( 'NONE',  ( -16.16747268278624716, -40.42849113817944584, -16.49999999999999645 ) ) ;
#4480=DIRECTION ( 'NONE',  ( -0.000000000000000000, -0.000000000000000000, -1.000000000000000000 ) ) ;
#4486=CARTESIAN_POINT ( 'NONE',  ( 21.14511335159655658, -37.62126931545598296, -16.50000000000000000 ) ) ;
#4489=DIRECTION ( 'NONE',  ( 1.000000000000000000, 0.000000000000000000, 0.000000000000000000 ) ) ;
#4493=ORIENTED_EDGE ( 'NONE', *, *, #2912, .T. ) ;
#4504=PLANE ( 'NONE',  #22888 ) ;
#4542=CARTESIAN_POINT ( 'NONE',  ( -11.30959556923743392, 42.34504995199416300, -16.50000000000000000 ) ) ;
#4556=CARTESIAN_POINT ( 'NONE',  ( 20.65888525914559892, 38.75220717792412728, -19.50000000000000355 ) ) ;
#4557=DIRECTION ( 'NONE',  ( -1.000000000000000000, 0.000000000000000000, 0.000000000000000000 ) ) ;
#4575=CARTESIAN_POINT ( 'NONE',  ( -19.64114023396299302, -37.13592150529018454, -1.500000000000000000 ) ) ;
#4583=ADVANCED_FACE ( 'NONE', ( #2215 ), #26228, .T. ) ;
#4586=DIRECTION ( 'NONE',  ( 0.5503133621338236470, 0.8349582046168341209, 0.000000000000000000 ) ) ;
#4589=DIRECTION ( 'NONE',  ( -0.06975647374412530244, 0.000000000000000000, -0.9975640502598241977 ) ) ;
#4608=CARTESIAN_POINT ( 'NONE',  ( -5.374868878254082105, 44.10336124695542992, -19.50000000000000355 ) ) ;
#4623=ORIENTED_EDGE ( 'NONE', *, *, #6175, .F. ) ;
#4634=CARTESIAN_POINT ( 'NONE',  ( 18.92760511682993751, -39.00287852246747633, -16.50000000000000711 ) ) ;
#4641=EDGE_CURVE ( 'NONE', #4182, #14649, #15809, .T. ) ;
#4642=EDGE_CURVE ( 'NONE', #4182, #15053, #16558, .T. ) ;
#4656=ORIENTED_EDGE ( 'NONE', *, *, #27078, .F. ) ;
#4657=LINE ( 'NONE', #18417, #16309 ) ;
#4666=EDGE_CURVE ( 'NONE', #19456, #8889, #26030, .T. ) ;
#4673=FACE_OUTER_BOUND ( 'NONE', #9260, .T. ) ;
#4678=CARTESIAN_POINT ( 'NONE',  ( 40.05104235265675783, 2.353288714459732311, -11.49999999999999645 ) ) ;
#4694=CARTESIAN_POINT ( 'NONE',  ( -25.64627119138473788, 23.40052582045089480, -6.500000000000000888 ) ) ;
#4695=CARTESIAN_POINT ( 'NONE',  ( -0.5234333628969437546, 44.07381280400610279, -16.50000000000000711 ) ) ;
#4701=EDGE_CURVE ( 'NONE', #2298, #17387, #7332, .T. ) ;
#4705=CARTESIAN_POINT ( 'NONE',  ( 26.80246859415415273, 7.028748154183637631, -1.499999999999999556 ) ) ;
#4709=CARTESIAN_POINT ( 'NONE',  ( 39.83602371822922095, -11.57901747687539640, -19.50000000000000355 ) ) ;
#4728=ORIENTED_EDGE ( 'NONE', *, *, #9371, .F. ) ;
#4754=CARTESIAN_POINT ( 'NONE',  ( -12.56641067637617759, -40.32935944494947478, -1.500000000000000000 ) ) ;
#4760=ORIENTED_EDGE ( 'NONE', *, *, #8795, .T. ) ;
#4762=CARTESIAN_POINT ( 'NONE',  ( -32.93066663369632607, -23.11087908566834770, -3.166603007242238643 ) ) ;
#4777=ADVANCED_FACE ( 'NONE', ( #1116 ), #10784, .F. ) ;
#4827=CARTESIAN_POINT ( 'NONE',  ( 39.52380524535330153, 7.028748154198969367, -11.49999999999999645 ) ) ;
#4828=CARTESIAN_POINT ( 'NONE',  ( 23.28555253867649810, -23.03920922976760721, -16.50001200000000168 ) ) ;
#4831=FACE_OUTER_BOUND ( 'NONE', #2557, .T. ) ;
#4850=CARTESIAN_POINT ( 'NONE',  ( -10.31606103249976059, 42.64332891061493314, -16.49999999999999645 ) ) ;
#4860=CARTESIAN_POINT ( 'NONE',  ( -30.26724724044810699, -27.72993536917633151, -6.500000000000001776 ) ) ;
#4865=CARTESIAN_POINT ( 'NONE',  ( 4.336808689942017736E-16, 42.50000000000000000, -1.500000000000000000 ) ) ;
#4874=CARTESIAN_POINT ( 'NONE',  ( 39.83602371822922095, -11.57901747687539640, -19.50000000000000355 ) ) ;
#4884=CARTESIAN_POINT ( 'NONE',  ( -37.98493438988128901, 11.12428508575241004, -1.500000000000000000 ) ) ;
#4885=DIRECTION ( 'NONE',  ( -1.000000000000000000, 0.000000000000000000, 0.000000000000000000 ) ) ;
#4901=DIRECTION ( 'NONE',  ( 0.000000000000000000, -0.000000000000000000, -1.000000000000000000 ) ) ;
#4905=AXIS2_PLACEMENT_3D ( 'NONE', #19903, #1181, #29259 ) ;
#4906=CARTESIAN_POINT ( 'NONE',  ( 26.80246859415415273, 7.028748154183637631, -1.499999999999999556 ) ) ;
#4912=CARTESIAN_POINT ( 'NONE',  ( 5.105024945673418912, -42.22604126506271882, -1.500000000000000000 ) ) ;
#4916=CARTESIAN_POINT ( 'NONE',  ( -23.96732207939035675, 33.98584080153585774, -1.500000000000000000 ) ) ;
#4946=DIRECTION ( 'NONE',  ( -0.9547931052914335748, 0.2972711322815276835, 0.000000000000000000 ) ) ;
#4959=EDGE_CURVE ( 'NONE', #7694, #20319, #145, .T. ) ;
#4967=ORIENTED_EDGE ( 'NONE', *, *, #18387, .F. ) ;
#4968=LINE ( 'NONE', #2478, #10342 ) ;
#4972=VERTEX_POINT ( 'NONE', #28541 ) ;
#4991=CARTESIAN_POINT ( 'NONE',  ( -39.87350638640939593, 4.706224724266459880, -11.49999999999999645 ) ) ;
#5010=APPLICATION_CONTEXT ( 'automotive_design' ) ;
#5019=VERTEX_POINT ( 'NONE', #26627 ) ;
#5021=CARTESIAN_POINT ( 'NONE',  ( -23.96732207938974213, -33.98584080153308662, -1.500000000000000000 ) ) ;
#5030=CARTESIAN_POINT ( 'NONE',  ( -12.56641067637752229, 40.32935944495016400, -1.500000000000000000 ) ) ;
#5055=ORIENTED_EDGE ( 'NONE', *, *, #28673, .F. ) ;
#5057=CARTESIAN_POINT ( 'NONE',  ( 23.22298177387596141, 35.92225147269209629, -14.83329744754546375 ) ) ;
#5074=CARTESIAN_POINT ( 'NONE',  ( 35.76344986163714168, -22.29344514668044752, -19.50000000000000355 ) ) ;
#5092=CARTESIAN_POINT ( 'NONE',  ( 21.14235806497239167, 37.62311247503154021, -16.49999999999999645 ) ) ;
#5118=CARTESIAN_POINT ( 'NONE',  ( 31.61046531696969808, 26.43913157123721192, -9.833326301035395289 ) ) ;
#5122=ORIENTED_EDGE ( 'NONE', *, *, #4218, .F. ) ;
#5140=DIRECTION ( 'NONE',  ( 0.4539545692076743522, 0.8910248307962438385, -0.000000000000000000 ) ) ;
#5168=CARTESIAN_POINT ( 'NONE',  ( -1.734723475976807094E-15, -44.07656352898514740, -6.500000000000000888 ) ) ;
#5175=CARTESIAN_POINT ( 'NONE',  ( 10.11202017158399968, 41.14070756921128691, -1.500000000000000000 ) ) ;
#5185=CARTESIAN_POINT ( 'NONE',  ( -10.11202017158235833, -41.14070756921188377, -1.500000000000000000 ) ) ;
#5191=CARTESIAN_POINT ( 'NONE',  ( 33.78553947564427773, -24.40792753551981775, -16.50000000000000000 ) ) ;
#5205=CARTESIAN_POINT ( 'NONE',  ( -25.47847050916411504, 26.57182937991348481, -6.499999999999999112 ) ) ;
#5209=CARTESIAN_POINT ( 'NONE',  ( -21.37787209074186734, 24.17206580633116175, -16.50001200000000168 ) ) ;
#5211=CARTESIAN_POINT ( 'NONE',  ( 23.05654803991950175, 35.38768971483871439, -9.833278432202751773 ) ) ;
#5220=DIRECTION ( 'NONE',  ( -0.000000000000000000, -0.000000000000000000, -1.000000000000000000 ) ) ;
#5227=LINE ( 'NONE', #14433, #24389 ) ;
#5241=ADVANCED_FACE ( 'NONE', ( #25046 ), #6022, .F. ) ;
#5247=CARTESIAN_POINT ( 'NONE',  ( 19.81910295759737295, 38.46425637429425848, -16.50000000000000711 ) ) ;
#5270=CARTESIAN_POINT ( 'NONE',  ( 32.08353429860093797, 26.68014822794475549, -14.83332872293874871 ) ) ;
#5297=CARTESIAN_POINT ( 'NONE',  ( 24.03057240117691862, 26.57182937991349903, -16.50000000000000000 ) ) ;
#5302=ORIENTED_EDGE ( 'NONE', *, *, #22477, .F. ) ;
#5312=CARTESIAN_POINT ( 'NONE',  ( -33.14492814497880602, 23.43596551657908122, -6.499906363187105462 ) ) ;
#5313=VECTOR ( 'NONE', #19564, 1000.000000000000000 ) ;
#5321=AXIS2_PLACEMENT_3D ( 'NONE', #11971, #19592, #26624 ) ;
#5329=CARTESIAN_POINT ( 'NONE',  ( -40.89187623478217404, 5.790488632116478129, -19.50000000000000355 ) ) ;
#5330=DIRECTION ( 'NONE',  ( 0.000000000000000000, -1.000000000000000000, 0.000000000000000000 ) ) ;
#5331=ORIENTED_EDGE ( 'NONE', *, *, #6695, .F. ) ;
#5336=CARTESIAN_POINT ( 'NONE',  ( 23.96732207937828463, 33.98584080152456011, -1.500000000000000000 ) ) ;
#5350=AXIS2_PLACEMENT_3D ( 'NONE', #2827, #29029, #26538 ) ;
#5404=CARTESIAN_POINT ( 'NONE',  ( 22.58267429318971864, 26.57182937991349903, 26.54355021145563143 ) ) ;
#5421=AXIS2_PLACEMENT_3D ( 'NONE', #28656, #22083, #2922 ) ;
#5438=VERTEX_POINT ( 'NONE', #30342 ) ;
#5444=CARTESIAN_POINT ( 'NONE',  ( 32.08353429544116864, -26.68014823150863890, -14.83332872412183789 ) ) ;
#5479=CYLINDRICAL_SURFACE ( 'NONE', #313, 1.447898107987198646 ) ;
#5481=CARTESIAN_POINT ( 'NONE',  ( 24.03057240117691862, 26.57182937991349903, -1.500000000000001332 ) ) ;
#5497=CARTESIAN_POINT ( 'NONE',  ( -5.374868878256215510, -44.10336124695545124, -19.50000000000000355 ) ) ;
#5528=CARTESIAN_POINT ( 'NONE',  ( 2.687479363073301819, 44.39187623479102740, -19.50000000000000355 ) ) ;
#5532=ORIENTED_EDGE ( 'NONE', *, *, #22201, .F. ) ;
#5533=FACE_OUTER_BOUND ( 'NONE', #22627, .T. ) ;
#5564=EDGE_CURVE ( 'NONE', #25162, #2292, #1475, .T. ) ;
#5571=VERTEX_POINT ( 'NONE', #13326 ) ;
#5573=EDGE_CURVE ( 'NONE', #752, #30725, #10663, .T. ) ;
#5641=CARTESIAN_POINT ( 'NONE',  ( -31.29501345865529061, -26.27841684422010360, -6.500000000000000888 ) ) ;
#5653=CARTESIAN_POINT ( 'NONE',  ( -34.07766914599908148, -21.40380666528021081, -1.500000000000000000 ) ) ;
#5660=FACE_OUTER_BOUND ( 'NONE', #19726, .T. ) ;
#5662=ORIENTED_EDGE ( 'NONE', *, *, #22148, .T. ) ;
#5671=CARTESIAN_POINT ( 'NONE',  ( -20.48466473087059470, 26.10042409808303887, -16.50001200000000168 ) ) ;
#5681=CARTESIAN_POINT ( 'NONE',  ( -10.64374042650306862, 42.96126232887723972, -19.50000000000000355 ) ) ;
#5686=CARTESIAN_POINT ( 'NONE',  ( -12.56641067637617759, -40.32935944494947478, -1.500000000000000000 ) ) ;
#5694=EDGE_LOOP ( 'NONE', ( #6793, #18652, #23579, #22900, #7663 ) ) ;
#5709=CARTESIAN_POINT ( 'NONE',  ( -40.56315269328749196, 1.166124675481670092, -16.50000000000000000 ) ) ;
#5718=ORIENTED_EDGE ( 'NONE', *, *, #1153, .T. ) ;
#5728=DIRECTION ( 'NONE',  ( 0.4539545692076743522, -0.8910248307962438385, 0.000000000000000000 ) ) ;
#5758=CIRCLE ( 'NONE', #29174, 1.447898107987198646 ) ;
#5769=ADVANCED_FACE ( 'NONE', ( #19208 ), #12944, .T. ) ;
#5780=EDGE_CURVE ( 'NONE', #12085, #477, #29622, .T. ) ;
#5795=DIRECTION ( 'NONE',  ( 0.000000000000000000, -0.000000000000000000, -1.000000000000000000 ) ) ;
#5816=ORIENTED_EDGE ( 'NONE', *, *, #27689, .F. ) ;
#5827=AXIS2_PLACEMENT_3D ( 'NONE', #24997, #18294, #15956 ) ;
#5840=CARTESIAN_POINT ( 'NONE',  ( 39.83602371822922095, -11.57901747687539640, -19.50000000000000355 ) ) ;
#5846=CARTESIAN_POINT ( 'NONE',  ( 34.07766914600081520, 21.40380666527109810, -1.500000000000000000 ) ) ;
#5851=CARTESIAN_POINT ( 'NONE',  ( 13.22505861668195237, -42.10773672056998862, -19.50000000000000355 ) ) ;
#5869=CARTESIAN_POINT ( 'NONE',  ( -40.57398644816432665, 0.5759020631866372808, -16.50000000000000000 ) ) ;
#5884=VECTOR ( 'NONE', #28837, 1000.000000000000000 ) ;
#5885=DIRECTION ( 'NONE',  ( -0.000000000000000000, -0.000000000000000000, -1.000000000000000000 ) ) ;
#5910=DIRECTION ( 'NONE',  ( 0.000000000000000000, -1.000000000000000000, 0.000000000000000000 ) ) ;
#5912=CYLINDRICAL_SURFACE ( 'NONE', #28244, 3.559164065751841743 ) ;
#5972=ORIENTED_EDGE ( 'NONE', *, *, #22924, .F. ) ;
#5977=VERTEX_POINT ( 'NONE', #23965 ) ;
#5978=LINE ( 'NONE', #3022, #15867 ) ;
#5994=CARTESIAN_POINT ( 'NONE',  ( -5.374868878254082105, 44.10336124695542992, -19.50000000000000355 ) ) ;
#5999=CARTESIAN_POINT ( 'NONE',  ( -23.96732207938974213, -33.98584080153308662, -1.500000000000000000 ) ) ;
#6002=ORIENTED_EDGE ( 'NONE', *, *, #28246, .F. ) ;
#6003=VECTOR ( 'NONE', #981, 1000.000000000000000 ) ;
#6005=CARTESIAN_POINT ( 'NONE',  ( -2.687479362164884034, -44.39187623478217404, -19.50000000000000355 ) ) ;
#6009=VERTEX_POINT ( 'NONE', #21152 ) ;
#6022=PLANE ( 'NONE',  #30766 ) ;
#6023=DIRECTION ( 'NONE',  ( -0.000000000000000000, -0.000000000000000000, -1.000000000000000000 ) ) ;
#6031=B_SPLINE_CURVE_WITH_KNOTS ( 'NONE', 3,
 ( #6500, #11029, #22870, #10876, #11182, #18203, #1362 ),
 .UNSPECIFIED., .F., .F.,
 ( 4, 3, 4 ),
 ( 0.000000000000000000, 0.005031266823827981044, 0.01006253384101580411 ),
 .UNSPECIFIED. ) ;
#6033=CARTESIAN_POINT ( 'NONE',  ( 32.74775157611827581, 27.21557300921217859, -19.50000000000000355 ) ) ;
#6088=DIRECTION ( 'NONE',  ( 1.000000000000000000, -0.000000000000000000, -0.000000000000000000 ) ) ;
#6136=LINE ( 'NONE', #25011, #13791 ) ;
#6142=CARTESIAN_POINT ( 'NONE',  ( -40.89187623478217404, 5.790488632116478129, -19.50000000000000355 ) ) ;
#6147=CARTESIAN_POINT ( 'NONE',  ( -13.22505861668333083, 42.10773672057167261, -19.50000000000000355 ) ) ;
#6153=CARTESIAN_POINT ( 'NONE',  ( -20.65888525914364493, -38.75220717792906555, -19.50000000000000355 ) ) ;
#6163=ORIENTED_EDGE ( 'NONE', *, *, #28673, .T. ) ;
#6175=EDGE_CURVE ( 'NONE', #22154, #544, #7758, .T. ) ;
#6177=DIRECTION ( 'NONE',  ( -1.000000000000000000, 0.000000000000000000, 0.000000000000000000 ) ) ;
#6193=CARTESIAN_POINT ( 'NONE',  ( -33.78553900464347493, 24.40792682089791654, -16.50000000000000000 ) ) ;
#6227=CARTESIAN_POINT ( 'NONE',  ( -12.33859880789484365, 8.132258305203428961, -16.50000000000000000 ) ) ;
#6249=ORIENTED_EDGE ( 'NONE', *, *, #19476, .F. ) ;
#6254=VERTEX_POINT ( 'NONE', #10237 ) ;
#6268=CARTESIAN_POINT ( 'NONE',  ( 39.87350638640939593, 4.706224724266460768, -6.500000000000000888 ) ) ;
#6276=CARTESIAN_POINT ( 'NONE',  ( -23.27838112031802709, -36.10018649381529343, -16.50000600000000262 ) ) ;
#6294=CARTESIAN_POINT ( 'NONE',  ( -39.00000000000000000, -5.563236990218529243, -1.500000000000000000 ) ) ;
#6295=CARTESIAN_POINT ( 'NONE',  ( -23.16753609997193664, 35.74416776803685281, -13.16661218272965783 ) ) ;
#6299=CARTESIAN_POINT ( 'NONE',  ( -2.552544030762004645, -42.50000000000000000, -1.500000000000000000 ) ) ;
#6305=CARTESIAN_POINT ( 'NONE',  ( 13.22505861668094340, 42.10773672057246841, -19.50000000000000355 ) ) ;
#6313=CARTESIAN_POINT ( 'NONE',  ( 23.27838111857050407, -36.10018641471199174, -16.50000599999999906 ) ) ;
#6314=VECTOR ( 'NONE', #9388, 1000.000000000000000 ) ;
#6320=ORIENTED_EDGE ( 'NONE', *, *, #1153, .F. ) ;
#6331=EDGE_CURVE ( 'NONE', #20319, #2261, #20670, .T. ) ;
#6335=ORIENTED_EDGE ( 'NONE', *, *, #11073, .F. ) ;
#6336=EDGE_CURVE ( 'NONE', #7694, #26229, #6612, .T. ) ;
#6355=CARTESIAN_POINT ( 'NONE',  ( -1.045628782875250185, -44.07656352898515451, -16.50000000000000000 ) ) ;
#6370=DIRECTION ( 'NONE',  ( -0.000000000000000000, -0.000000000000000000, -1.000000000000000000 ) ) ;
#6406=ADVANCED_FACE ( 'NONE', ( #7101 ), #4459, .F. ) ;
#6410=CARTESIAN_POINT ( 'NONE',  ( 30.26724724045341119, 27.72993536918018265, -6.500000000000000888 ) ) ;
#6419=PRODUCT_DEFINITION_FORMATION_WITH_SPECIFIED_SOURCE ( 'ANY', '', #21363, .NOT_KNOWN. ) ;
#6452=EDGE_LOOP ( 'NONE', ( #10370, #3859, #2915, #19681 ) ) ;
#6467=ORIENTED_EDGE ( 'NONE', *, *, #5564, .T. ) ;
#6468=CARTESIAN_POINT ( 'NONE',  ( -39.83602371821034183, 11.57901747687032490, -19.50000000000000355 ) ) ;
#6477=LINE ( 'NONE', #8814, #27739 ) ;
#6478=FACE_OUTER_BOUND ( 'NONE', #30530, .T. ) ;
#6485=CARTESIAN_POINT ( 'NONE',  ( 31.29501345866090389, 26.27841684422296353, -6.500000000000000888 ) ) ;
#6491=CARTESIAN_POINT ( 'NONE',  ( 35.78163722268750746, -27.43648963448195133, -1.500000000000000000 ) ) ;
#6496=CARTESIAN_POINT ( 'NONE',  ( 5.374868878254059013, -44.10336124695543703, -19.50000000000000355 ) ) ;
#6500=CARTESIAN_POINT ( 'NONE',  ( 22.94541271838008356, -35.03073867843704647, -6.500000000000000888 ) ) ;
#6510=EDGE_CURVE ( 'NONE', #2261, #2130, #9175, .T. ) ;
#6514=AXIS2_PLACEMENT_3D ( 'NONE', #2012, #13575, #13717 ) ;
#6528=FACE_OUTER_BOUND ( 'NONE', #14522, .T. ) ;
#6603=CARTESIAN_POINT ( 'NONE',  ( 19.64114023396309960, -37.13592150529014191, -1.500000000000000000 ) ) ;
#6604=CARTESIAN_POINT ( 'NONE',  ( 40.89187623478217404, 5.790488632116406187, -19.50000000000000355 ) ) ;
#6609=CARTESIAN_POINT ( 'NONE',  ( -10.11202017158466759, 41.14070756921185534, -1.500000000000000000 ) ) ;
#6612=CIRCLE ( 'NONE', #2127, 27.70876437800068359 ) ;
#6623=CARTESIAN_POINT ( 'NONE',  ( -31.29501345865439532, 26.27841684421964885, -6.500000000000000888 ) ) ;
#6642=CARTESIAN_POINT ( 'NONE',  ( -19.64114023396061981, 37.13592150528867109, -1.500000000000000000 ) ) ;
#6644=ORIENTED_EDGE ( 'NONE', *, *, #11651, .F. ) ;
#6652=CARTESIAN_POINT ( 'NONE',  ( -21.14806837890567692, -37.61929654846579041, -16.50000000000000000 ) ) ;
#6662=B_SPLINE_SURFACE_WITH_KNOTS ( 'NONE', 1, 3, ( 
 ( #22826, #5528, #22661, #29868, #13020, #25160, #29547, #13328, #8509, #8181, #27204, #8341, #5840, #1311, #15497, #10667, #17537, #27056, #10989, #25015, #1477, #10829, #30010, #15339, #20338, #12711, #27521, #12872, #10366, #24870, #24545, #6142, #22371, #1156, #20173, #8651, #17856, #27373, #5681, #5994, #3806, #18159 ),
 ( #15029, #3191, #844, #22208, #8033, #19880, #24697, #3340, #29695, #28284, #6750, #27974, #9410, #30155, #11445, #8955, #6603, #3969, #27665, #15968, #16119, #25488, #20931, #4414, #4111, #23276, #25638, #30308, #21082, #22972, #6294, #16265, #30602, #23577, #9246, #15806, #1629, #11140, #25326, #18471, #4254, #18766 ) ),
 .UNSPECIFIED., .F., .T., .F.,
 ( 2, 2 ),
 ( 4, 2, 2, 2, 2, 2, 2, 2, 2, 2, 2, 2, 2, 2, 2, 2, 2, 2, 2, 2, 4 ),
 ( 0.000000000000000000, 1.000000000000000000 ),
 ( 0.000000000000000000, 0.1963495408493620697, 0.3926990816987241395, 0.7853981633974482790, 1.178097245096172418, 1.570796326794896558, 1.963495408493620697, 2.356194490192344837, 2.748893571891068976, 2.945243112740430824, 3.141592653589793116, 3.337942194439155408, 3.534291735288517255, 3.926990816987241395, 4.319689898685965090, 4.712388980384689674, 5.105088062083414258, 5.497787143782137953, 5.890486225480861648, 6.086835766330223940, 6.283185307179586232 ),
 .UNSPECIFIED. ) ;
#6674=VERTEX_POINT ( 'NONE', #12239 ) ;
#6695=EDGE_CURVE ( 'NONE', #22584, #8392, #16637, .T. ) ;
#6696=DIRECTION ( 'NONE',  ( -1.000000000000000000, 0.000000000000000000, 0.000000000000000000 ) ) ;
#6706=ORIENTED_EDGE ( 'NONE', *, *, #10099, .F. ) ;
#6714=EDGE_CURVE ( 'NONE', #12583, #23101, #8652, .T. ) ;
#6730=CARTESIAN_POINT ( 'NONE',  ( -8.304834736901785419, 43.14465394274145638, -16.50000000000000355 ) ) ;
#6750=CARTESIAN_POINT ( 'NONE',  ( 39.00000000000000000, 5.563236990218597633, -1.500000000000000000 ) ) ;
#6751=CARTESIAN_POINT ( 'NONE',  ( 5.374868878255610660, 44.10336124695606230, -19.50000000000000355 ) ) ;
#6752=ORIENTED_EDGE ( 'NONE', *, *, #16434, .F. ) ;
#6755=CARTESIAN_POINT ( 'NONE',  ( -2.552544031601109875, 42.50000000001772094, -1.500000000000000000 ) ) ;
#6757=CARTESIAN_POINT ( 'NONE',  ( 25.23756106473024019, 11.43858098102958287, -1.500000000000000000 ) ) ;
#6760=CARTESIAN_POINT ( 'NONE',  ( -12.56641067637617759, -40.32935944494947478, -1.500000000000000000 ) ) ;
#6774=LINE ( 'NONE', #17603, #29066 ) ;
#6783=DIRECTION ( 'NONE',  ( -1.000000000000000000, 0.000000000000000000, 0.000000000000000000 ) ) ;
#6791=CARTESIAN_POINT ( 'NONE',  ( 4.336808689942017736E-16, 42.50000000000000000, -1.500000000000000000 ) ) ;
#6793=ORIENTED_EDGE ( 'NONE', *, *, #4185, .T. ) ;
#6802=CARTESIAN_POINT ( 'NONE',  ( -9.792086282299422351, -42.77788222952042929, -16.50000000000000355 ) ) ;
#6837=VERTEX_POINT ( 'NONE', #13782 ) ;
#6846=CARTESIAN_POINT ( 'NONE',  ( 20.47140833542507821, -26.57182937991349903, -6.500000000000000888 ) ) ;
#6853=VERTEX_POINT ( 'NONE', #25933 ) ;
#6857=AXIS2_PLACEMENT_3D ( 'NONE', #16480, #19434, #9617 ) ;
#6860=ORIENTED_EDGE ( 'NONE', *, *, #15116, .T. ) ;
#6878=ORIENTED_EDGE ( 'NONE', *, *, #13585, .F. ) ;
#6883=CARTESIAN_POINT ( 'NONE',  ( -0.2599583092368172865, 44.07656244530785727, -16.50000000000000355 ) ) ;
#6909=ADVANCED_FACE ( 'NONE', ( #9411 ), #13136, .T. ) ;
#6911=CARTESIAN_POINT ( 'NONE',  ( 25.19442432474404470, 35.44676296256560022, -19.50000000000000355 ) ) ;
#6933=DIRECTION ( 'NONE',  ( 0.2972711322815261292, 0.9547931052914340189, 0.000000000000000000 ) ) ;
#6936=ORIENTED_EDGE ( 'NONE', *, *, #30002, .F. ) ;
#6949=CARTESIAN_POINT ( 'NONE',  ( -24.03057240117691862, -26.57182937991349903, -6.500000000000000888 ) ) ;
#6970=ORIENTED_EDGE ( 'NONE', *, *, #4666, .T. ) ;
#6978=CARTESIAN_POINT ( 'NONE',  ( 21.79579286733899579, -37.18345238509958506, -16.49999999999999645 ) ) ;
#6980=VECTOR ( 'NONE', #21201, 1000.000000000000000 ) ;
#6982=PLANE ( 'NONE',  #25503 ) ;
#6988=ORIENTED_EDGE ( 'NONE', *, *, #21940, .T. ) ;
#7019=VERTEX_POINT ( 'NONE', #15461 ) ;
#7021=CARTESIAN_POINT ( 'NONE',  ( -19.64114023396061981, 37.13592150528867109, -1.500000000000009992 ) ) ;
#7038=VERTEX_POINT ( 'NONE', #20598 ) ;
#7048=DIRECTION ( 'NONE',  ( -1.000000000000000000, 0.000000000000000000, 0.000000000000000000 ) ) ;
#7049=B_SPLINE_CURVE_WITH_KNOTS ( 'NONE', 3,
 ( #26222, #4860, #14374, #16872, #2527, #9691 ),
 .UNSPECIFIED., .F., .F.,
 ( 4, 2, 4 ),
 ( 0.001794032523744105035, 0.007046146517947431132, 0.01388807892444383733 ),
 .UNSPECIFIED. ) ;
#7050=CARTESIAN_POINT ( 'NONE',  ( -25.19442432475839055, 35.44676296258369064, -19.50000000000000355 ) ) ;
#7051=CARTESIAN_POINT ( 'NONE',  ( 24.03057240117691862, 26.57182937991349903, -1.500000000000001332 ) ) ;
#7087=LINE ( 'NONE', #19092, #17815 ) ;
#7093=LINE ( 'NONE', #4906, #9399 ) ;
#7099=VECTOR ( 'NONE', #1512, 1000.000000000000114 ) ;
#7101=FACE_OUTER_BOUND ( 'NONE', #7291, .T. ) ;
#7105=CARTESIAN_POINT ( 'NONE',  ( -5.105024945675580739, -42.22604126506273303, -1.500000000000000000 ) ) ;
#7113=EDGE_CURVE ( 'NONE', #13970, #2231, #24075, .T. ) ;
#7119=DIRECTION ( 'NONE',  ( -1.000000000000000000, 0.000000000000000000, 0.000000000000000000 ) ) ;
#7127=CARTESIAN_POINT ( 'NONE',  ( -23.96732207938974213, -33.98584080153308662, -1.500000000000000000 ) ) ;
#7145=ORIENTED_EDGE ( 'NONE', *, *, #9213, .F. ) ;
#7176=CARTESIAN_POINT ( 'NONE',  ( 20.47140923013457936, -25.96617498784419098, -16.50001200000000168 ) ) ;
#7188=ORIENTED_EDGE ( 'NONE', *, *, #7969, .F. ) ;
#7201=ORIENTED_EDGE ( 'NONE', *, *, #21993, .T. ) ;
#7203=CARTESIAN_POINT ( 'NONE',  ( 12.56641067637628240, -40.32935944494942504, -1.500000000000000000 ) ) ;
#7220=ORIENTED_EDGE ( 'NONE', *, *, #28234, .T. ) ;
#7233=CARTESIAN_POINT ( 'NONE',  ( 23.11204207310333203, 35.56592875157961231, -11.49994540239372043 ) ) ;
#7248=ORIENTED_EDGE ( 'NONE', *, *, #18369, .T. ) ;
#7265=CARTESIAN_POINT ( 'NONE',  ( -10.29532059365457108, -42.63824274976927597, -16.49999999999999645 ) ) ;
#7291=EDGE_LOOP ( 'NONE', ( #19300, #5972, #16929, #4728, #29965, #15753, #7700 ) ) ;
#7332=CIRCLE ( 'NONE', #349, 3.559164065751841743 ) ;
#7354=ADVANCED_FACE ( 'NONE', ( #4831 ), #7793, .T. ) ;
#7357=EDGE_CURVE ( 'NONE', #12085, #18281, #21830, .T. ) ;
#7369=CARTESIAN_POINT ( 'NONE',  ( -10.11202017158235833, -41.14070756921188377, -1.500000000000000000 ) ) ;
#7375=CARTESIAN_POINT ( 'NONE',  ( -33.78553900464347493, 24.40792682089791654, -16.50000000000000000 ) ) ;
#7378=CARTESIAN_POINT ( 'NONE',  ( -31.18700685316050780, 26.11823559932051353, -1.500000000000000000 ) ) ;
#7396=AXIS2_PLACEMENT_3D ( 'NONE', #9486, #28514, #21014 ) ;
#7417=CARTESIAN_POINT ( 'NONE',  ( 40.89187623478217404, 5.790488632116406187, -19.50000000000000355 ) ) ;
#7429=DIRECTION ( 'NONE',  ( -1.000000000000000000, 0.000000000000000000, 0.000000000000000000 ) ) ;
#7439=CARTESIAN_POINT ( 'NONE',  ( 1.038391619697657475, 44.07656847656198806, -16.49999999999999645 ) ) ;
#7450=ORIENTED_EDGE ( 'NONE', *, *, #27898, .F. ) ;
#7452=B_SPLINE_CURVE_WITH_KNOTS ( 'NONE', 3,
 ( #16489, #26006, #1989, #12229, #19405, #6978, #4486, #28923, #4634, #14134, #30380, #11513, #20996, #17056, #2870, #25546, #12394, #4169, #13699, #24071, #13995, #23493, #2135, #14714, #11652, #21143, #21728 ),
 .UNSPECIFIED., .F., .F.,
 ( 4, 2, 1, 1, 2, 2, 2, 2, 1, 1, 1, 2, 2, 2, 2, 4 ),
 ( 0.9060794618157798075, 0.9075469702249081561, 0.9090144786340366156, 0.9119494954522934238, 0.9178195290888072622, 0.9295595963618348279, 0.9530397309078899593, 0.9545072393170184188, 0.9559747477261468784, 0.9589097645444037976, 0.9647797981809175250, 0.9677148149991744441, 0.9706498318174312523, 0.9765198654539450906, 0.9882599327269725453, 1.000000000000000000 ),
 .UNSPECIFIED. ) ;
#7453=VECTOR ( 'NONE', #11108, 1000.000000000000000 ) ;
#7511=CARTESIAN_POINT ( 'NONE',  ( 20.47140833542507821, 26.57182937991349903, -6.500000000000000888 ) ) ;
#7512=DIRECTION ( 'NONE',  ( -1.000000000000000000, 0.000000000000000000, 0.000000000000000000 ) ) ;
#7520=PLANE ( 'NONE',  #3940 ) ;
#7526=CARTESIAN_POINT ( 'NONE',  ( -5.374868878254082105, 44.10336124695542992, -19.50000000000000355 ) ) ;
#7534=CARTESIAN_POINT ( 'NONE',  ( 2.552544030762014415, -42.50000000000000000, -1.500000000000000000 ) ) ;
#7564=DIRECTION ( 'NONE',  ( 0.000000000000000000, -0.000000000000000000, 1.000000000000000000 ) ) ;
#7566=CARTESIAN_POINT ( 'NONE',  ( 25.47847050916410439, -26.57182937991349903, -6.499999999999999112 ) ) ;
#7575=AXIS2_PLACEMENT_3D ( 'NONE', #16796, #4946, #13853 ) ;
#7585=B_SPLINE_CURVE_WITH_KNOTS ( 'NONE', 3,
 ( #22927, #24810, #24964, #13588, #20133, #27620 ),
 .UNSPECIFIED., .F., .F.,
 ( 4, 2, 4 ),
 ( 1.408367944312347353, 1.570796326794896558, 1.733224709277445319 ),
 .UNSPECIFIED. ) ;
#7590=CARTESIAN_POINT ( 'NONE',  ( 4.770489558936219510E-15, -42.50000000000000000, -1.500000000000000000 ) ) ;
#7616=CARTESIAN_POINT ( 'NONE',  ( 40.22758167353954661, -5.871156286330812435, -16.50000000000000711 ) ) ;
#7645=CARTESIAN_POINT ( 'NONE',  ( -32.08353429858341599, -26.68014822793582752, -14.83332872282386816 ) ) ;
#7661=CARTESIAN_POINT ( 'NONE',  ( -33.57242512142387625, 24.08458161877161885, -13.16663720014219408 ) ) ;
#7663=ORIENTED_EDGE ( 'NONE', *, *, #30002, .T. ) ;
#7677=CARTESIAN_POINT ( 'NONE',  ( 23.96732207938043402, -33.98584080152387088, -1.500000000000000000 ) ) ;
#7685=FACE_OUTER_BOUND ( 'NONE', #8037, .T. ) ;
#7687=CARTESIAN_POINT ( 'NONE',  ( 12.56641067637329812, 40.32935944495179115, -1.500000000000000000 ) ) ;
#7694=VERTEX_POINT ( 'NONE', #15184 ) ;
#7697=CARTESIAN_POINT ( 'NONE',  ( 2.168404344971008868E-16, 42.50000000000000711, -1.500000000000000000 ) ) ;
#7699=ORIENTED_EDGE ( 'NONE', *, *, #18925, .T. ) ;
#7700=ORIENTED_EDGE ( 'NONE', *, *, #26912, .F. ) ;
#7710=EDGE_CURVE ( 'NONE', #23836, #5438, #14730, .T. ) ;
#7723=CYLINDRICAL_SURFACE ( 'NONE', #23731, 3.559164065751841743 ) ;
#7730=CARTESIAN_POINT ( 'NONE',  ( 20.65888525914559892, 38.75220717792412728, -19.50000000000000355 ) ) ;
#7745=CARTESIAN_POINT ( 'NONE',  ( 13.27321688587731607, 41.66719137602760981, -16.50000000000000000 ) ) ;
#7747=EDGE_LOOP ( 'NONE', ( #11188, #21880, #13512, #15472 ) ) ;
#7758=LINE ( 'NONE', #24737, #18061 ) ;
#7793=CYLINDRICAL_SURFACE ( 'NONE', #22586, 27.70876437800068359 ) ;
#7814=CARTESIAN_POINT ( 'NONE',  ( 24.03057240117690441, -26.57182937991349903, 26.54355021145563143 ) ) ;
#7819=AXIS2_PLACEMENT_3D ( 'NONE', #16301, #18958, #24078 ) ;
#7833=CARTESIAN_POINT ( 'NONE',  ( 35.78163722268750746, -27.43648963448195133, -11.49999999999999645 ) ) ;
#7835=CARTESIAN_POINT ( 'NONE',  ( -13.22505861668184046, -42.10773672057003125, -19.50000000000000355 ) ) ;
#7841=CARTESIAN_POINT ( 'NONE',  ( 33.03787114092997257, -23.27353420009123042, -4.833239141675072403 ) ) ;
#7851=VERTEX_POINT ( 'NONE', #27674 ) ;
#7867=VECTOR ( 'NONE', #21453, 1000.000000000000114 ) ;
#7871=VECTOR ( 'NONE', #30378, 1000.000000000000000 ) ;
#7884=CARTESIAN_POINT ( 'NONE',  ( 2.687479363073301819, 44.39187623479102740, -19.50000000000000355 ) ) ;
#7922=AXIS2_PLACEMENT_3D ( 'NONE', #21935, #2766, #24430 ) ;
#7930=EDGE_CURVE ( 'NONE', #18437, #3296, #29876, .T. ) ;
#7937=CARTESIAN_POINT ( 'NONE',  ( 40.05520465696179855, -7.028746455191999587, -16.50000000000000000 ) ) ;
#7945=CARTESIAN_POINT ( 'NONE',  ( -25.47847050916411504, 26.57182937991348481, 26.54355021145563143 ) ) ;
#7949=AXIS2_PLACEMENT_3D ( 'NONE', #23239, #9069, #27640 ) ;
#7969=EDGE_CURVE ( 'NONE', #15053, #5977, #14070, .T. ) ;
#7997=EDGE_LOOP ( 'NONE', ( #10287, #29351, #25224, #11377 ) ) ;
#8001=CARTESIAN_POINT ( 'NONE',  ( -10.64374042650075403, -42.96126232887726815, -19.50000000000000355 ) ) ;
#8017=DIRECTION ( 'NONE',  ( -1.000000000000000000, 0.000000000000000000, 0.000000000000000000 ) ) ;
#8021=CARTESIAN_POINT ( 'NONE',  ( -21.14898501148481813, 24.45236287589831292, -16.50001200000000523 ) ) ;
#8026=DIRECTION ( 'NONE',  ( 1.000000000000000000, 0.000000000000000000, 0.000000000000000000 ) ) ;
#8033=CARTESIAN_POINT ( 'NONE',  ( 12.56641067637329812, 40.32935944495179115, -1.500000000000000000 ) ) ;
#8037=EDGE_LOOP ( 'NONE', ( #15704, #14677, #26407, #12702 ) ) ;
#8048=VERTEX_POINT ( 'NONE', #6757 ) ;
#8070=VECTOR ( 'NONE', #27589, 1000.000000000000000 ) ;
#8091=CARTESIAN_POINT ( 'NONE',  ( 39.52380524533145945, -7.028748154382054913, -11.49999999999999645 ) ) ;
#8095=FACE_OUTER_BOUND ( 'NONE', #7747, .T. ) ;
#8111=AXIS2_PLACEMENT_3D ( 'NONE', #5481, #14828, #17015 ) ;
#8171=DIRECTION ( 'NONE',  ( -0.5503133621338236470, -0.8349582046168341209, 0.000000000000000000 ) ) ;
#8181=CARTESIAN_POINT ( 'NONE',  ( 39.83602371821015709, 11.57901747687536265, -19.50000000000000355 ) ) ;
#8182=DIRECTION ( 'NONE',  ( 0.000000000000000000, -1.000000000000000000, 0.000000000000000000 ) ) ;
#8186=CARTESIAN_POINT ( 'NONE',  ( 39.00000000000000000, -5.563236990218592304, -1.500000000000000000 ) ) ;
#8192=CARTESIAN_POINT ( 'NONE',  ( 0.000000000000000000, 44.39187623478217404, -19.50000000000000355 ) ) ;
#8210=CARTESIAN_POINT ( 'NONE',  ( -40.22764886168826592, -5.870704729722422854, -16.50000000000000000 ) ) ;
#8211=DIRECTION ( 'NONE',  ( -0.8349582046168341209, 0.5503133621338236470, 0.000000000000000000 ) ) ;
#8223=CARTESIAN_POINT ( 'NONE',  ( -32.74775157610760346, -27.21557300919352329, -19.50000000000000355 ) ) ;
#8225=ORIENTED_EDGE ( 'NONE', *, *, #24838, .T. ) ;
#8242=DIRECTION ( 'NONE',  ( -0.000000000000000000, -0.000000000000000000, -1.000000000000000000 ) ) ;
#8283=CIRCLE ( 'NONE', #1308, 7.500000000000000000 ) ;
#8296=DIRECTION ( 'NONE',  ( -1.000000000000000000, 0.000000000000000000, 0.000000000000000000 ) ) ;
#8299=DIRECTION ( 'NONE',  ( -0.000000000000000000, -0.000000000000000000, -1.000000000000000000 ) ) ;
#8341=CARTESIAN_POINT ( 'NONE',  ( 40.89187623478217404, -5.790488632116400858, -19.50000000000000355 ) ) ;
#8346=CARTESIAN_POINT ( 'NONE',  ( -10.64374042650075403, -42.96126232887726815, -19.50000000000000355 ) ) ;
#8348=DIRECTION ( 'NONE',  ( -0.000000000000000000, -0.000000000000000000, 1.000000000000000000 ) ) ;
#8352=CARTESIAN_POINT ( 'NONE',  ( 10.11202017158399968, 41.14070756921128691, -1.500000000000000000 ) ) ;
#8356=B_SPLINE_CURVE_WITH_KNOTS ( 'NONE', 3,
 ( #4385, #1605, #2195, #27644, #6268, #18591 ),
 .UNSPECIFIED., .F., .F.,
 ( 4, 2, 4 ),
 ( 1.408367944307647113, 1.570796326794821507, 1.733224709277370712 ),
 .UNSPECIFIED. ) ;
#8377=ORIENTED_EDGE ( 'NONE', *, *, #24212, .F. ) ;
#8383=CARTESIAN_POINT ( 'NONE',  ( 20.65888525914559892, 38.75220717792412728, -19.50000000000000355 ) ) ;
#8388=ADVANCED_BREP_SHAPE_REPRESENTATION ( '', ( #2654, #7396 ), #14351 ) ;
#8392=VERTEX_POINT ( 'NONE', #9502 ) ;
#8413=CARTESIAN_POINT ( 'NONE',  ( 0.000000000000000000, 0.000000000000000000, -11.49999999999999645 ) ) ;
#8502=EDGE_CURVE ( 'NONE', #26952, #16888, #25402, .T. ) ;
#8509=CARTESIAN_POINT ( 'NONE',  ( 35.76344986165623396, 22.29344514668041199, -19.50000000000000355 ) ) ;
#8514=CARTESIAN_POINT ( 'NONE',  ( -37.98493438988128901, 11.12428508575241004, -1.500000000000000000 ) ) ;
#8516=CARTESIAN_POINT ( 'NONE',  ( 12.33859880789482233, -8.132258305203423632, -16.50000000000000000 ) ) ;
#8518=AXIS2_PLACEMENT_3D ( 'NONE', #23827, #21485, #9336 ) ;
#8520=CARTESIAN_POINT ( 'NONE',  ( -5.374868878254082105, 44.10336124695542992, -19.50000000000000355 ) ) ;
#8544=CARTESIAN_POINT ( 'NONE',  ( 39.83602371822922095, -11.57901747687539640, -19.50000000000000355 ) ) ;
#8571=VERTEX_POINT ( 'NONE', #10907 ) ;
#8592=CIRCLE ( 'NONE', #25508, 7.500000000000000000 ) ;
#8594=ORIENTED_EDGE ( 'NONE', *, *, #17172, .T. ) ;
#8605=LINE ( 'NONE', #20587, #30656 ) ;
#8615=ADVANCED_FACE ( 'NONE', ( #30831 ), #261, .T. ) ;
#8623=ORIENTED_EDGE ( 'NONE', *, *, #28658, .T. ) ;
#8634=CARTESIAN_POINT ( 'NONE',  ( -24.27860874716793660, -23.00333360197815935, -16.50001199999999812 ) ) ;
#8637=LINE ( 'NONE', #3797, #29048 ) ;
#8644=ADVANCED_FACE ( 'NONE', ( #9628, #16647 ), #6982, .T. ) ;
#8646=VECTOR ( 'NONE', #9194, 1000.000000000000000 ) ;
#8651=CARTESIAN_POINT ( 'NONE',  ( -25.19442432475839055, 35.44676296258369064, -19.50000000000000355 ) ) ;
#8652=LINE ( 'NONE', #30156, #12608 ) ;
#8655=CARTESIAN_POINT ( 'NONE',  ( -5.374868878254082105, 44.10336124695542992, -19.50000000000000355 ) ) ;
#8658=ORIENTED_EDGE ( 'NONE', *, *, #9213, .T. ) ;
#8704=CARTESIAN_POINT ( 'NONE',  ( 39.52380524535562500, 7.028748154183637631, -11.49999999999999645 ) ) ;
#8737=EDGE_LOOP ( 'NONE', ( #19098, #14560, #3012, #8658 ) ) ;
#8749=DIRECTION ( 'NONE',  ( -0.000000000000000000, -0.000000000000000000, 1.000000000000000000 ) ) ;
#8768=EDGE_LOOP ( 'NONE', ( #3510, #21833, #11526, #25676 ) ) ;
#8776=DIRECTION ( 'NONE',  ( -0.000000000000000000, -0.000000000000000000, -1.000000000000000000 ) ) ;
#8792=CARTESIAN_POINT ( 'NONE',  ( 5.105024945673418912, -42.22604126506271882, -1.500000000000000000 ) ) ;
#8795=EDGE_CURVE ( 'NONE', #25580, #19866, #23348, .T. ) ;
#8801=CARTESIAN_POINT ( 'NONE',  ( -10.64374042650075403, -42.96126232887726815, -19.50000000000000355 ) ) ;
#8814=CARTESIAN_POINT ( 'NONE',  ( 20.71335220384823117, 27.86167394782616213, -6.500000000000000888 ) ) ;
#8818=ADVANCED_FACE ( 'NONE', ( #27279 ), #5912, .F. ) ;
#8822=B_SPLINE_CURVE_WITH_KNOTS ( 'NONE', 3,
 ( #6276, #3637, #27651, #25623, #15788, #27814, #13312 ),
 .UNSPECIFIED., .F., .F.,
 ( 4, 3, 4 ),
 ( 0.000000000000000000, 0.005031266826610968426, 0.01006253384379828669 ),
 .UNSPECIFIED. ) ;
#8851=CARTESIAN_POINT ( 'NONE',  ( -5.720368925487725242, -43.64004031045374887, -16.49999999999999645 ) ) ;
#8857=ADVANCED_FACE ( 'NONE', ( #28471 ), #7723, .F. ) ;
#8865=DIRECTION ( 'NONE',  ( -1.000000000000000000, 0.000000000000000000, 0.000000000000000000 ) ) ;
#8866=LINE ( 'NONE', #4025, #23241 ) ;
#8868=B_SPLINE_CURVE_WITH_KNOTS ( 'NONE', 3,
 ( #2496, #28860, #19030, #12165 ),
 .UNSPECIFIED., .F., .F.,
 ( 4, 4 ),
 ( 0.000000000000000000, 0.005028157979160191408 ),
 .UNSPECIFIED. ) ;
#8876=EDGE_CURVE ( 'NONE', #2425, #20269, #4332, .T. ) ;
#8889=VERTEX_POINT ( 'NONE', #26595 ) ;
#8892=ORIENTED_EDGE ( 'NONE', *, *, #19283, .F. ) ;
#8893=DIRECTION ( 'NONE',  ( -1.000000000000000000, 0.000000000000000000, 0.000000000000000000 ) ) ;
#8916=EDGE_CURVE ( 'NONE', #14001, #12141, #21902, .T. ) ;
#8949=ORIENTED_EDGE ( 'NONE', *, *, #10730, .T. ) ;
#8955=CARTESIAN_POINT ( 'NONE',  ( 23.96732207938043402, -33.98584080152387088, -1.500000000000000000 ) ) ;
#8957=CARTESIAN_POINT ( 'NONE',  ( 25.19442432473618254, -35.44676296258426618, -19.50000000000000355 ) ) ;
#8966=DIRECTION ( 'NONE',  ( -0.000000000000000000, -0.000000000000000000, -1.000000000000000000 ) ) ;
#8982=ADVANCED_FACE ( 'NONE', ( #14580 ), #29694, .F. ) ;
#8995=CARTESIAN_POINT ( 'NONE',  ( 5.105024945673418912, -42.22604126506271882, -1.500000000000000000 ) ) ;
#9016=LINE ( 'NONE', #23182, #326 ) ;
#9069=DIRECTION ( 'NONE',  ( -0.000000000000000000, -0.000000000000000000, 1.000000000000000000 ) ) ;
#9085=CARTESIAN_POINT ( 'NONE',  ( -5.729465025513086419E-13, 44.07656359094158915, -16.50000000000000000 ) ) ;
#9108=CARTESIAN_POINT ( 'NONE',  ( 4.336808689942017736E-16, 42.50000000000000000, -1.500000000000000000 ) ) ;
#9116=ORIENTED_EDGE ( 'NONE', *, *, #29177, .F. ) ;
#9135=CARTESIAN_POINT ( 'NONE',  ( -10.11202017158235833, -41.14070756921188377, -1.500000000000000000 ) ) ;
#9147=CARTESIAN_POINT ( 'NONE',  ( -33.14492811172277698, -23.43596546612170073, -6.499905845449016617 ) ) ;
#9149=CARTESIAN_POINT ( 'NONE',  ( -11.79670489141087231, -42.17678086688154337, -16.49999999999999645 ) ) ;
#9154=EDGE_CURVE ( 'NONE', #6837, #24446, #1847, .T. ) ;
#9157=ORIENTED_EDGE ( 'NONE', *, *, #12817, .T. ) ;
#9175=B_SPLINE_CURVE_WITH_KNOTS ( 'NONE', 3,
 ( #2254, #14104, #18806, #16758, #30490, #19252, #26274, #4912, #21592, #226 ),
 .UNSPECIFIED., .F., .F.,
 ( 4, 2, 2, 2, 4 ),
 ( 0.2152766488939568124, 0.2238273688332776123, 0.2394469624395233198, 0.2472567592426461458, 0.2550665560457689995 ),
 .UNSPECIFIED. ) ;
#9179=DIRECTION ( 'NONE',  ( -0.9547931052914339078, -0.2972711322815266843, 0.000000000000000000 ) ) ;
#9183=LINE ( 'NONE', #18244, #15474 ) ;
#9191=ORIENTED_EDGE ( 'NONE', *, *, #18906, .F. ) ;
#9194=DIRECTION ( 'NONE',  ( -0.000000000000000000, -0.000000000000000000, -1.000000000000000000 ) ) ;
#9196=EDGE_CURVE ( 'NONE', #26952, #12085, #20306, .T. ) ;
#9204=ORIENTED_EDGE ( 'NONE', *, *, #455, .T. ) ;
#9213=EDGE_CURVE ( 'NONE', #13938, #11031, #19776, .T. ) ;
#9225=CARTESIAN_POINT ( 'NONE',  ( -5.729465025513086419E-13, 44.07656359094158915, -16.50000000000000000 ) ) ;
#9229=CARTESIAN_POINT ( 'NONE',  ( -7.500000000000000000, 0.000000000000000000, 63.50000000000000000 ) ) ;
#9246=CARTESIAN_POINT ( 'NONE',  ( -31.18700685316050780, 26.11823559932051353, -1.500000000000000000 ) ) ;
#9258=CARTESIAN_POINT ( 'NONE',  ( -10.11202017158235833, -41.14070756921188377, -1.500000000000000000 ) ) ;
#9260=EDGE_LOOP ( 'NONE', ( #10277, #2016, #7450, #26967, #7699, #24982, #6335 ) ) ;
#9280=DIRECTION ( 'NONE',  ( 0.000000000000000000, 0.000000000000000000, -1.000000000000000000 ) ) ;
#9288=CARTESIAN_POINT ( 'NONE',  ( -31.18700685316100163, -26.11823559932341610, -1.500000000000000000 ) ) ;
#9298=CARTESIAN_POINT ( 'NONE',  ( -16.40045772880338859, -40.31754624252415198, -16.50000000000000000 ) ) ;
#9319=CIRCLE ( 'NONE', #25751, 1.447898107987198646 ) ;
#9328=AXIS2_PLACEMENT_3D ( 'NONE', #1757, #8776, #18605 ) ;
#9336=DIRECTION ( 'NONE',  ( 0.06975647374412530244, 0.000000000000000000, -0.9975640502598241977 ) ) ;
#9339=DIRECTION ( 'NONE',  ( -0.000000000000000000, -0.000000000000000000, 1.000000000000000000 ) ) ;
#9345=LINE ( 'NONE', #16206, #17127 ) ;
#9353=ADVANCED_FACE ( 'NONE', ( #16688 ), #3937, .F. ) ;
#9371=EDGE_CURVE ( 'NONE', #15207, #3753, #8868, .T. ) ;
#9378=CARTESIAN_POINT ( 'NONE',  ( -26.80246859415415273, 7.028748154183637631, -6.500000000000000888 ) ) ;
#9380=ADVANCED_FACE ( 'NONE', ( #16988 ), #21664, .T. ) ;
#9386=ORIENTED_EDGE ( 'NONE', *, *, #26582, .T. ) ;
#9388=DIRECTION ( 'NONE',  ( -0.000000000000000000, -0.000000000000000000, -1.000000000000000000 ) ) ;
#9390=CARTESIAN_POINT ( 'NONE',  ( 33.78553947564427773, -24.40792753551981775, -16.50000000000000000 ) ) ;
#9392=LINE ( 'NONE', #19367, #11821 ) ;
#9396=ORIENTED_EDGE ( 'NONE', *, *, #25397, .T. ) ;
#9399=VECTOR ( 'NONE', #12233, 1000.000000000000000 ) ;
#9401=CARTESIAN_POINT ( 'NONE',  ( -39.83602371821034183, 11.57901747687032490, -19.50000000000000355 ) ) ;
#9406=B_SPLINE_CURVE_WITH_KNOTS ( 'NONE', 3,
 ( #28159, #11951, #30640, #28328, #20829, #30803, #14255, #21442, #1812, #25525 ),
 .UNSPECIFIED., .F., .F.,
 ( 4, 3, 3, 4 ),
 ( 3.702578198638058010E-17, 0.005033946524314943105, 0.01006789357361646473, 0.01510156516273209251 ),
 .UNSPECIFIED. ) ;
#9410=CARTESIAN_POINT ( 'NONE',  ( 37.98493438989863336, -11.12428508576153341, -1.500000000000000000 ) ) ;
#9411=FACE_OUTER_BOUND ( 'NONE', #27646, .T. ) ;
#9413=ORIENTED_EDGE ( 'NONE', *, *, #4641, .T. ) ;
#9442=B_SPLINE_CURVE_WITH_KNOTS ( 'NONE', 3,
 ( #3604, #25588, #18431, #1111, #6410, #4065 ),
 .UNSPECIFIED., .F., .F.,
 ( 4, 2, 4 ),
 ( 0.001913784325927354304, 0.008754285094829554470, 0.01400530011240105378 ),
 .UNSPECIFIED. ) ;
#9445=DIRECTION ( 'NONE',  ( -0.000000000000000000, -0.000000000000000000, -1.000000000000000000 ) ) ;
#9453=CARTESIAN_POINT ( 'NONE',  ( -2.552544030762004645, -42.50000000000000000, -1.500000000000000000 ) ) ;
#9467=FACE_OUTER_BOUND ( 'NONE', #14620, .T. ) ;
#9468=DIRECTION ( 'NONE',  ( -1.000000000000000000, 0.000000000000000000, 0.000000000000000000 ) ) ;
#9486=CARTESIAN_POINT ( 'NONE',  ( 0.000000000000000000, 0.000000000000000000, 0.000000000000000000 ) ) ;
#9487=EDGE_LOOP ( 'NONE', ( #4656, #23510, #4493, #3129 ) ) ;
#9497=ORIENTED_EDGE ( 'NONE', *, *, #23837, .T. ) ;
#9502=CARTESIAN_POINT ( 'NONE',  ( -23.27838111883973227, 36.10018642694448943, -16.50000600000000262 ) ) ;
#9510=CARTESIAN_POINT ( 'NONE',  ( 25.23756106473024730, -11.43858098102957577, -11.49999999999999645 ) ) ;
#9529=CARTESIAN_POINT ( 'NONE',  ( -8.809276947023224835, 43.02645599243116692, -16.50000000000000000 ) ) ;
#9544=CARTESIAN_POINT ( 'NONE',  ( 5.374868878254059013, -44.10336124695543703, -19.50000000000000355 ) ) ;
#9554=ORIENTED_EDGE ( 'NONE', *, *, #29982, .T. ) ;
#9562=CARTESIAN_POINT ( 'NONE',  ( 23.96732207938043402, -33.98584080152387088, -1.500000000000000000 ) ) ;
#9591=VECTOR ( 'NONE', #27381, 1000.000000000000114 ) ;
#9616=ORIENTED_EDGE ( 'NONE', *, *, #17172, .F. ) ;
#9617=DIRECTION ( 'NONE',  ( 1.000000000000000000, 0.000000000000000000, 0.000000000000000000 ) ) ;
#9620=CARTESIAN_POINT ( 'NONE',  ( 22.43462709106480091, 36.72607276382733943, -16.50000000000000000 ) ) ;
#9626=APPLICATION_CONTEXT ( 'automotive_design' ) ;
#9628=FACE_BOUND ( 'NONE', #16581, .T. ) ;
#9634=ORIENTED_EDGE ( 'NONE', *, *, #7969, .T. ) ;
#9635=ORIENTED_EDGE ( 'NONE', *, *, #22101, .F. ) ;
#9640=( LENGTH_UNIT ( ) NAMED_UNIT ( * ) SI_UNIT ( .MILLI., .METRE. ) );
#9669=CARTESIAN_POINT ( 'NONE',  ( -40.05104235265675783, -2.353288714459718989, -6.500000000000000888 ) ) ;
#9678=ORIENTED_EDGE ( 'NONE', *, *, #13983, .F. ) ;
#9683=CARTESIAN_POINT ( 'NONE',  ( -2.616297575292053423, 43.98845571999485315, -16.50000000000000000 ) ) ;
#9690=FACE_BOUND ( 'NONE', #28964, .T. ) ;
#9691=CARTESIAN_POINT ( 'NONE',  ( -22.94541271838176755, -35.03073867844241818, -6.500000000000000888 ) ) ;
#9695=CARTESIAN_POINT ( 'NONE',  ( -35.76344986165604212, -22.29344514668547461, -19.50000000000000355 ) ) ;
#9703=CARTESIAN_POINT ( 'NONE',  ( 31.18700685317242716, 26.11823559933198879, -1.500000000000000000 ) ) ;
#9744=CARTESIAN_POINT ( 'NONE',  ( 35.76344986165623396, 22.29344514668041199, -19.50000000000000355 ) ) ;
#9766=CARTESIAN_POINT ( 'NONE',  ( 23.07173088127199279, 36.25735992984930789, -16.49999999999999645 ) ) ;
#9779=ADVANCED_FACE ( 'NONE', ( #20509, #6478 ), #1335, .F. ) ;
#9837=PLANE ( 'NONE',  #21276 ) ;
#9842=CARTESIAN_POINT ( 'NONE',  ( -32.82330813384395185, 22.94799032727105370, -1.500000000000000000 ) ) ;
#9845=ORIENTED_EDGE ( 'NONE', *, *, #19075, .T. ) ;
#9849=CARTESIAN_POINT ( 'NONE',  ( -33.13218612630368654, -7.028748154183637631, -1.942616967526160643 ) ) ;
#9857=CARTESIAN_POINT ( 'NONE',  ( -5.374868878256215510, -44.10336124695545124, -19.50000000000000355 ) ) ;
#9859=ORIENTED_EDGE ( 'NONE', *, *, #20240, .T. ) ;
#9865=CARTESIAN_POINT ( 'NONE',  ( 2.552544031601107211, 42.49999999998228617, -1.500000000000000000 ) ) ;
#9870=CARTESIAN_POINT ( 'NONE',  ( 33.57242512144424751, -24.08458161880252035, -13.16663720046962638 ) ) ;
#9873=CARTESIAN_POINT ( 'NONE',  ( -32.24119442679361214, -26.76047168400493703, -16.50000600000000262 ) ) ;
#9888=CARTESIAN_POINT ( 'NONE',  ( 2.552544031601107211, 42.49999999998228617, -1.500000000000003997 ) ) ;
#9924=CARTESIAN_POINT ( 'NONE',  ( -22.58267429318971864, 26.57182937991348481, 26.54355021145563143 ) ) ;
#9925=AXIS2_PLACEMENT_3D ( 'NONE', #19381, #17348, #3007 ) ;
#9926=CARTESIAN_POINT ( 'NONE',  ( 20.26334714462845099, 38.18989983590572024, -16.50000000000000355 ) ) ;
#9937=CARTESIAN_POINT ( 'NONE',  ( 33.16313691975489064, 7.028748154183637631, -1.500000000000000000 ) ) ;
#9961=ORIENTED_EDGE ( 'NONE', *, *, #22707, .T. ) ;
#9979=EDGE_CURVE ( 'NONE', #16888, #477, #17747, .T. ) ;
#9998=DIRECTION ( 'NONE',  ( 0.9547931052914340189, -0.2972711322815261292, 0.000000000000000000 ) ) ;
#10016=CARTESIAN_POINT ( 'NONE',  ( 31.18700685317242716, 26.11823559933198879, -1.500000000000000000 ) ) ;
#10023=CARTESIAN_POINT ( 'NONE',  ( -2.552544031601109875, 42.50000000001772094, -1.500000000000000000 ) ) ;
#10059=CARTESIAN_POINT ( 'NONE',  ( 0.000000000000000000, 44.39187623478217404, -19.50000000000000355 ) ) ;
#10068=CARTESIAN_POINT ( 'NONE',  ( -33.67904611720921793, -24.24635140548038237, -14.83330431372253777 ) ) ;
#10074=CARTESIAN_POINT ( 'NONE',  ( -19.64114023396299302, -37.13592150529018454, -1.500000000000000000 ) ) ;
#10079=FACE_BOUND ( 'NONE', #434, .T. ) ;
#10099=EDGE_CURVE ( 'NONE', #2298, #29282, #25002, .T. ) ;
#10128=ADVANCED_FACE ( 'NONE', ( #18146 ), #15484, .F. ) ;
#10168=CARTESIAN_POINT ( 'NONE',  ( -35.76344986165608475, 22.29344514668535027, -19.50000000000000355 ) ) ;
#10173=EDGE_LOOP ( 'NONE', ( #10576, #4623, #30126, #19213 ) ) ;
#10176=CARTESIAN_POINT ( 'NONE',  ( -33.53985809055312473, -24.80926221883534311, -16.50000000000000355 ) ) ;
#10184=ORIENTED_EDGE ( 'NONE', *, *, #2891, .F. ) ;
#10218=DIRECTION ( 'NONE',  ( -0.000000000000000000, -0.000000000000000000, 1.000000000000000000 ) ) ;
#10234=FACE_OUTER_BOUND ( 'NONE', #12497, .T. ) ;
#10237=CARTESIAN_POINT ( 'NONE',  ( 20.71335220384823472, 27.86167394782616924, -16.50000000000000000 ) ) ;
#10240=ORIENTED_EDGE ( 'NONE', *, *, #12253, .F. ) ;
#10251=CARTESIAN_POINT ( 'NONE',  ( 40.22845766574619830, 5.865279063056531683, -16.50000000000000000 ) ) ;
#10269=EDGE_CURVE ( 'NONE', #26065, #2425, #8866, .T. ) ;
#10277=ORIENTED_EDGE ( 'NONE', *, *, #20457, .F. ) ;
#10286=CARTESIAN_POINT ( 'NONE',  ( -31.92585768968024595, -26.59981599184672518, -13.16665969293629423 ) ) ;
#10287=ORIENTED_EDGE ( 'NONE', *, *, #24013, .F. ) ;
#10305=CARTESIAN_POINT ( 'NONE',  ( 31.29501345866090389, 26.27841684422296353, -6.500000000000000888 ) ) ;
#10315=CARTESIAN_POINT ( 'NONE',  ( -12.56641067637752229, 40.32935944495016400, -1.500000000000000000 ) ) ;
#10324=CARTESIAN_POINT ( 'NONE',  ( 39.00000000000000000, 5.563236990218597633, -1.500000000000000000 ) ) ;
#10342=VECTOR ( 'NONE', #443, 1000.000000000000000 ) ;
#10351=CARTESIAN_POINT ( 'NONE',  ( -20.58367780861512841, 27.52817754551177032, -16.50001200000000168 ) ) ;
#10366=CARTESIAN_POINT ( 'NONE',  ( -35.76344986165604212, -22.29344514668547461, -19.50000000000000355 ) ) ;
#10370=ORIENTED_EDGE ( 'NONE', *, *, #23180, .T. ) ;
#10399=CARTESIAN_POINT ( 'NONE',  ( -40.48935727530044915, 2.936718089577218915, -16.50000000000000355 ) ) ;
#10491=CARTESIAN_POINT ( 'NONE',  ( 25.64627119138473432, -23.40052582045089480, -16.50000000000000000 ) ) ;
#10514=FACE_OUTER_BOUND ( 'NONE', #17944, .T. ) ;
#10520=CARTESIAN_POINT ( 'NONE',  ( -5.374868878256215510, -44.10336124695545124, -19.50000000000000355 ) ) ;
#10524=DIRECTION ( 'NONE',  ( 0.8910248307962433945, -0.4539545692076750738, 0.000000000000000000 ) ) ;
#10525=ORIENTED_EDGE ( 'NONE', *, *, #1052, .T. ) ;
#10530=ORIENTED_EDGE ( 'NONE', *, *, #2658, .F. ) ;
#10556=DIRECTION ( 'NONE',  ( -0.000000000000000000, -0.000000000000000000, 1.000000000000000000 ) ) ;
#10558=ORIENTED_EDGE ( 'NONE', *, *, #9371, .T. ) ;
#10560=CARTESIAN_POINT ( 'NONE',  ( -20.65888525914364493, -38.75220717792906555, -19.50000000000000355 ) ) ;
#10566=CARTESIAN_POINT ( 'NONE',  ( 0.000000000000000000, 0.000000000000000000, 63.50000000000000000 ) ) ;
#10576=ORIENTED_EDGE ( 'NONE', *, *, #29297, .F. ) ;
#10579=ORIENTED_EDGE ( 'NONE', *, *, #24597, .F. ) ;
#10598=CIRCLE ( 'NONE', #18567, 1.447898107987198646 ) ;
#10627=CARTESIAN_POINT ( 'NONE',  ( -37.98493438988128901, 11.12428508575241004, -1.500000000000000000 ) ) ;
#10628=DIRECTION ( 'NONE',  ( 0.000000000000000000, 0.000000000000000000, -1.000000000000000000 ) ) ;
#10658=FACE_OUTER_BOUND ( 'NONE', #21662, .T. ) ;
#10663=LINE ( 'NONE', #11136, #29005 ) ;
#10667=CARTESIAN_POINT ( 'NONE',  ( 25.19442432473618254, -35.44676296258426618, -19.50000000000000355 ) ) ;
#10672=CARTESIAN_POINT ( 'NONE',  ( 4.336808689942017736E-16, 42.50000000000000000, -1.500000000000000000 ) ) ;
#10677=CARTESIAN_POINT ( 'NONE',  ( -40.89187623478217404, 5.790488632116478129, -19.50000000000000355 ) ) ;
#10690=ORIENTED_EDGE ( 'NONE', *, *, #25460, .T. ) ;
#10692=DIRECTION ( 'NONE',  ( 0.8910248307962437275, 0.4539545692076742966, -0.000000000000000000 ) ) ;
#10697=CARTESIAN_POINT ( 'NONE',  ( -40.05520443301966083, -7.028746486913004077, -16.50000000000000000 ) ) ;
#10730=EDGE_CURVE ( 'NONE', #30328, #5571, #9319, .T. ) ;
#10784=PLANE ( 'NONE',  #24752 ) ;
#10804=EDGE_LOOP ( 'NONE', ( #6988, #15048, #22031, #709 ) ) ;
#10816=DIRECTION ( 'NONE',  ( -1.000000000000000000, 0.000000000000000000, 0.000000000000000000 ) ) ;
#10829=CARTESIAN_POINT ( 'NONE',  ( -2.687479362164884034, -44.39187623478217404, -19.50000000000000355 ) ) ;
#10836=CARTESIAN_POINT ( 'NONE',  ( -37.98493438988125348, -11.12428508575252728, -1.500000000000000000 ) ) ;
#10843=CARTESIAN_POINT ( 'NONE',  ( 32.74775157611827581, 27.21557300921217859, -19.50000000000000355 ) ) ;
#10850=FACE_OUTER_BOUND ( 'NONE', #24887, .T. ) ;
#10865=CARTESIAN_POINT ( 'NONE',  ( 25.64627119138473432, -23.40052582045089480, -6.500000000000000888 ) ) ;
#10876=CARTESIAN_POINT ( 'NONE',  ( 23.11204206675566297, -35.56592873119179643, -11.49994521172425976 ) ) ;
#10907=CARTESIAN_POINT ( 'NONE',  ( 32.82330813384650270, 22.94799032727486932, -1.500000000000000000 ) ) ;
#10931=FACE_OUTER_BOUND ( 'NONE', #25708, .T. ) ;
#10968=CARTESIAN_POINT ( 'NONE',  ( 32.24119409414369386, 26.76047229433004659, -16.50000600000000262 ) ) ;
#10972=CARTESIAN_POINT ( 'NONE',  ( 39.52380524533145945, -7.028748154382054913, -11.49999999999999645 ) ) ;
#10979=CARTESIAN_POINT ( 'NONE',  ( 25.64627119138473432, 23.40052582045089480, -6.500000000000000888 ) ) ;
#10989=CARTESIAN_POINT ( 'NONE',  ( 10.64374042650304020, -42.96126232887725394, -19.50000000000000355 ) ) ;
#10994=CARTESIAN_POINT ( 'NONE',  ( 31.18700685317242716, 26.11823559933198879, -1.500000000000000000 ) ) ;
#10999=CARTESIAN_POINT ( 'NONE',  ( -10.64374042650306862, 42.96126232887723972, -19.50000000000000355 ) ) ;
#11005=CARTESIAN_POINT ( 'NONE',  ( -32.08353430114796367, 26.68014822536797226, -14.83332872408068148 ) ) ;
#11025=EDGE_CURVE ( 'NONE', #6674, #14001, #8605, .T. ) ;
#11029=CARTESIAN_POINT ( 'NONE',  ( 23.00100564131886927, -35.20929533517521293, -8.166629612182571663 ) ) ;
#11031=VERTEX_POINT ( 'NONE', #1434 ) ;
#11073=EDGE_CURVE ( 'NONE', #7851, #25580, #14029, .T. ) ;
#11108=DIRECTION ( 'NONE',  ( 1.000000000000000000, 0.000000000000000000, 0.000000000000000000 ) ) ;
#11110=ORIENTED_EDGE ( 'NONE', *, *, #7113, .F. ) ;
#11123=CARTESIAN_POINT ( 'NONE',  ( -31.29501345865439532, 26.27841684421964885, -6.500000000000000888 ) ) ;
#11126=CARTESIAN_POINT ( 'NONE',  ( -25.32744450373244760, 23.23809170341762709, -16.50001200000000168 ) ) ;
#11136=CARTESIAN_POINT ( 'NONE',  ( -33.16313691975489064, -0.000000000000000000, -1.500000000000000000 ) ) ;
#11140=CARTESIAN_POINT ( 'NONE',  ( -12.56641067637752229, 40.32935944495016400, -1.500000000000000000 ) ) ;
#11141=CARTESIAN_POINT ( 'NONE',  ( -23.05654803568342359, 35.38768970123298629, -9.833278305020469290 ) ) ;
#11144=CARTESIAN_POINT ( 'NONE',  ( 37.98493438989863336, -11.12428508576153341, -1.500000000000000000 ) ) ;
#11150=CARTESIAN_POINT ( 'NONE',  ( -39.83602371821029919, -11.57901747687044924, -19.50000000000000355 ) ) ;
#11174=VERTEX_POINT ( 'NONE', #12955 ) ;
#11182=CARTESIAN_POINT ( 'NONE',  ( 23.16753609997519092, -35.74416776804734752, -13.16661218287092971 ) ) ;
#11188=ORIENTED_EDGE ( 'NONE', *, *, #13585, .T. ) ;
#11196=CARTESIAN_POINT ( 'NONE',  ( -39.52380524535903561, -7.028748154198949827, -6.500000000000000888 ) ) ;
#11222=CARTESIAN_POINT ( 'NONE',  ( -30.26724724044731829, 27.72993536917570623, -6.500000000000000888 ) ) ;
#11224=ORIENTED_EDGE ( 'NONE', *, *, #7710, .F. ) ;
#11259=ORIENTED_EDGE ( 'NONE', *, *, #28016, .T. ) ;
#11264=ORIENTED_EDGE ( 'NONE', *, *, #5780, .F. ) ;
#11270=CARTESIAN_POINT ( 'NONE',  ( -21.90865045291186775, -23.69204963285888610, -16.50001200000000168 ) ) ;
#11283=AXIS2_PLACEMENT_3D ( 'NONE', #21183, #19173, #14030 ) ;
#11289=CARTESIAN_POINT ( 'NONE',  ( 35.76344986163714168, -22.29344514668044752, -19.50000000000000355 ) ) ;
#11298=CARTESIAN_POINT ( 'NONE',  ( -20.71335220384823117, -27.86167394782616213, -16.50000000000000000 ) ) ;
#11322=CARTESIAN_POINT ( 'NONE',  ( 22.94541271838008356, -35.03073867843704647, -6.500000000000000888 ) ) ;
#11325=PLANE ( 'NONE',  #74 ) ;
#11326=CARTESIAN_POINT ( 'NONE',  ( 39.52380524533145945, -7.028748154382054913, -11.49999999999999645 ) ) ;
#11359=VECTOR ( 'NONE', #19130, 1000.000000000000000 ) ;
#11377=ORIENTED_EDGE ( 'NONE', *, *, #23145, .F. ) ;
#11389=CARTESIAN_POINT ( 'NONE',  ( -22.94541271838176044, 35.03073867844246081, -6.500000000000000888 ) ) ;
#11401=DIRECTION ( 'NONE',  ( -0.2972711322815274615, 0.9547931052914335748, -0.000000000000000000 ) ) ;
#11433=CARTESIAN_POINT ( 'NONE',  ( -20.48466473087059114, -26.10042409808303887, -16.50001200000000523 ) ) ;
#11445=CARTESIAN_POINT ( 'NONE',  ( 31.18700685317022803, -26.11823559933272421, -1.500000000000000000 ) ) ;
#11447=CARTESIAN_POINT ( 'NONE',  ( 10.64374042650304020, -42.96126232887725394, -19.50000000000000355 ) ) ;
#11457=CARTESIAN_POINT ( 'NONE',  ( -31.18700685316100163, -26.11823559932341610, -1.500000000000000000 ) ) ;
#11468=DIRECTION ( 'NONE',  ( 1.000000000000000000, 0.000000000000000000, 0.000000000000000000 ) ) ;
#11477=DIRECTION ( 'NONE',  ( -0.5503133621338236470, 0.8349582046168341209, -0.000000000000000000 ) ) ;
#11478=CARTESIAN_POINT ( 'NONE',  ( 40.05520465696179855, -7.028746455191999587, -16.50000000000000000 ) ) ;
#11485=ORIENTED_EDGE ( 'NONE', *, *, #21390, .F. ) ;
#11500=CARTESIAN_POINT ( 'NONE',  ( -20.27188091683318660, -38.18452458809359484, -16.50000000000000000 ) ) ;
#11513=CARTESIAN_POINT ( 'NONE',  ( 12.20512804738064716, -42.03592599325837398, -16.50000000000000355 ) ) ;
#11526=ORIENTED_EDGE ( 'NONE', *, *, #7930, .T. ) ;
#11535=CARTESIAN_POINT ( 'NONE',  ( -39.52380524536136619, -7.028748154183637631, -1.499999999999999556 ) ) ;
#11557=CARTESIAN_POINT ( 'NONE',  ( 2.168404344971008868E-16, 42.50000000000000711, -1.500000000000000000 ) ) ;
#11569=CARTESIAN_POINT ( 'NONE',  ( -5.221130439941095602, 43.71380105377362213, -16.49999999999999645 ) ) ;
#11572=CARTESIAN_POINT ( 'NONE',  ( -40.05104235265675783, -2.353288714454546238, -11.49999999999999645 ) ) ;
#11603=CARTESIAN_POINT ( 'NONE',  ( -33.78553900464347493, 24.40792682089791654, -16.50000000000000000 ) ) ;
#11622=CARTESIAN_POINT ( 'NONE',  ( -25.64627119138473432, -23.40052582045089480, -6.500000000000000888 ) ) ;
#11630=CARTESIAN_POINT ( 'NONE',  ( -20.65888525914099105, 38.75220717792564784, -19.50000000000000355 ) ) ;
#11638=CARTESIAN_POINT ( 'NONE',  ( -32.82330813384598400, -22.94799032726886523, -1.500000000000000000 ) ) ;
#11646=DIRECTION ( 'NONE',  ( 0.000000000000000000, 0.000000000000000000, -1.000000000000000000 ) ) ;
#11649=CARTESIAN_POINT ( 'NONE',  ( -40.05520497409654013, 7.028746409781321702, -16.50000000000000000 ) ) ;
#11651=EDGE_CURVE ( 'NONE', #29372, #25287, #30681, .T. ) ;
#11652=CARTESIAN_POINT ( 'NONE',  ( 2.095349214508610114, -44.03244755841715374, -16.50000000000000355 ) ) ;
#11672=CARTESIAN_POINT ( 'NONE',  ( -20.71335220384823117, 27.86167394782616213, -16.50001200000000168 ) ) ;
#11685=B_SPLINE_CURVE_WITH_KNOTS ( 'NONE', 3,
 ( #20083, #10251, #732, #29452, #22104, #3398, #17592, #12759, #19614, #15080, #12927, #17737, #7616, #7937 ),
 .UNSPECIFIED., .F., .F.,
 ( 4, 2, 1, 1, 2, 2, 2, 4 ),
 ( 0.7234904873890852794, 0.7367515904914523350, 0.7433821420426358628, 0.7466974178182276267, 0.7483550557060234532, 0.7500126935938193906, 0.7632737966961864462, 0.7765348997985535018 ),
 .UNSPECIFIED. ) ;
#11687=CYLINDRICAL_SURFACE ( 'NONE', #15577, 1.447898107987198646 ) ;
#11702=CARTESIAN_POINT ( 'NONE',  ( -23.96732207939035675, 33.98584080153585774, -1.500000000000009992 ) ) ;
#11716=VERTEX_POINT ( 'NONE', #21882 ) ;
#11719=EDGE_LOOP ( 'NONE', ( #24205, #8225, #21370, #9396 ) ) ;
#11731=CARTESIAN_POINT ( 'NONE',  ( -12.56641067637617759, -40.32935944494947478, -1.500000000000000000 ) ) ;
#11739=CARTESIAN_POINT ( 'NONE',  ( 5.374868878254059013, -44.10336124695543703, -19.50000000000000355 ) ) ;
#11741=CARTESIAN_POINT ( 'NONE',  ( -24.03057240117691862, 26.57182937991348481, -6.499999999999999112 ) ) ;
#11743=CARTESIAN_POINT ( 'NONE',  ( -31.18700685316050780, 26.11823559932051353, -1.500000000000000000 ) ) ;
#11749=CARTESIAN_POINT ( 'NONE',  ( -39.00000000000000000, 5.563236990218665134, -1.500000000000000000 ) ) ;
#11775=AXIS2_PLACEMENT_3D ( 'NONE', #8413, #16646, #4489 ) ;
#11779=CARTESIAN_POINT ( 'NONE',  ( 2.552544030762014415, -42.50000000000000000, -1.500000000000000000 ) ) ;
#11791=DIRECTION ( 'NONE',  ( 0.000000000000000000, 0.000000000000000000, -1.000000000000000000 ) ) ;
#11796=B_SPLINE_CURVE_WITH_KNOTS ( 'NONE', 3,
 ( #20537, #6355, #15868, #25385, #13540, #29751, #23020, #8851, #21131, #25683, #6802, #7265, #30817, #9149, #23626, #13839, #16326, #4477, #9298, #26294, #23947, #4307, #21610, #11500, #6652, #2270, #2594, #12112, #18664 ),
 .UNSPECIFIED., .F., .F.,
 ( 4, 1, 2, 2, 2, 2, 2, 2, 1, 2, 2, 1, 2, 2, 2, 4 ),
 ( 0.000000000000000000, 0.01176252312833788068, 0.01470315391042235215, 0.01764378469250681841, 0.02352504625667574054, 0.03528756938501358825, 0.04116883094918252078, 0.04705009251335146025, 0.05881261564168926981, 0.06175324642377374995, 0.06469387720585821622, 0.07057513877002716263, 0.07645640033419609516, 0.08233766189836502769, 0.08821892346253397410, 0.09410018502670292051 ),
 .UNSPECIFIED. ) ;
#11811=ORIENTED_EDGE ( 'NONE', *, *, #21993, .F. ) ;
#11821=VECTOR ( 'NONE', #17019, 1000.000000000000000 ) ;
#11831=CARTESIAN_POINT ( 'NONE',  ( 25.23756106473024730, -11.43858098102957577, -1.500000000000000000 ) ) ;
#11849=LINE ( 'NONE', #21346, #5884 ) ;
#11871=ORIENTED_EDGE ( 'NONE', *, *, #1976, .F. ) ;
#11885=CARTESIAN_POINT ( 'NONE',  ( -19.62486380000566655, 38.57793056412522503, -16.50000000000000000 ) ) ;
#11899=CARTESIAN_POINT ( 'NONE',  ( 35.76344986163714168, -22.29344514668044752, -19.50000000000000355 ) ) ;
#11901=CARTESIAN_POINT ( 'NONE',  ( 39.87808514715981545, 7.028748144847113188, -14.83333104077163256 ) ) ;
#11909=CARTESIAN_POINT ( 'NONE',  ( 0.000000000000000000, 44.39187623478217404, -19.50000000000000355 ) ) ;
#11920=CARTESIAN_POINT ( 'NONE',  ( -2.552544030762004645, -42.50000000000000000, -1.500000000000000000 ) ) ;
#11935=CARTESIAN_POINT ( 'NONE',  ( 10.11202017158399968, 41.14070756921128691, -1.500000000000003997 ) ) ;
#11951=CARTESIAN_POINT ( 'NONE',  ( 32.93066663369882718, 23.11087908567089855, -3.166603007242253298 ) ) ;
#11952=CARTESIAN_POINT ( 'NONE',  ( -31.18700685316050780, 26.11823559932051353, -1.500000000000000000 ) ) ;
#11963=CARTESIAN_POINT ( 'NONE',  ( 25.64627119138473432, -23.40052582045089480, -6.500000000000000888 ) ) ;
#11968=CARTESIAN_POINT ( 'NONE',  ( -29.55332031600282150, -27.89853503084716380, -1.500000000000000000 ) ) ;
#11971=CARTESIAN_POINT ( 'NONE',  ( 0.000000000000000000, 0.000000000000000000, -1.500000000000000000 ) ) ;
#11982=ORIENTED_EDGE ( 'NONE', *, *, #14536, .T. ) ;
#11999=CARTESIAN_POINT ( 'NONE',  ( -24.03057240117691862, 26.57182937991348481, 26.54355021145563143 ) ) ;
#12025=DIRECTION ( 'NONE',  ( 0.000000000000000000, 0.000000000000000000, -1.000000000000000000 ) ) ;
#12032=CARTESIAN_POINT ( 'NONE',  ( -22.86203465710450899, 36.41373663176752018, -16.50000000000000000 ) ) ;
#12039=CARTESIAN_POINT ( 'NONE',  ( 33.53985887099113228, -24.80926055130403896, -16.50000000000000000 ) ) ;
#12040=DIRECTION ( 'NONE',  ( -1.000000000000000000, -0.000000000000000000, -0.000000000000000000 ) ) ;
#12046=CARTESIAN_POINT ( 'NONE',  ( -13.22505861668333083, 42.10773672057167261, -19.50000000000000355 ) ) ;
#12055=CARTESIAN_POINT ( 'NONE',  ( 0.000000000000000000, 44.39187623478217404, -19.50000000000000355 ) ) ;
#12064=CARTESIAN_POINT ( 'NONE',  ( 7.500000000000000000, 9.184850993605147944E-16, -16.50000000000000000 ) ) ;
#12085=VERTEX_POINT ( 'NONE', #4694 ) ;
#12112=CARTESIAN_POINT ( 'NONE',  ( -22.86252527946696844, -36.41647737164041132, -16.50000000000000000 ) ) ;
#12118=CARTESIAN_POINT ( 'NONE',  ( 18.91580660644371292, 38.99778335661734729, -16.50000000000000000 ) ) ;
#12141=VERTEX_POINT ( 'NONE', #17320 ) ;
#12165=CARTESIAN_POINT ( 'NONE',  ( -39.52380524536136619, -7.028748154183644736, -11.49999999999999645 ) ) ;
#12180=EDGE_LOOP ( 'NONE', ( #8949, #19217 ) ) ;
#12194=CARTESIAN_POINT ( 'NONE',  ( 20.65888525914375862, -38.75220717792901581, -19.50000000000000355 ) ) ;
#12196=ORIENTED_EDGE ( 'NONE', *, *, #92, .T. ) ;
#12200=CARTESIAN_POINT ( 'NONE',  ( -40.89187623478217404, -5.790488632116337797, -19.50000000000000355 ) ) ;
#12213=VERTEX_POINT ( 'NONE', #22304 ) ;
#12225=ORIENTED_EDGE ( 'NONE', *, *, #5573, .T. ) ;
#12228=DIRECTION ( 'NONE',  ( -1.000000000000000000, 0.000000000000000000, 0.000000000000000000 ) ) ;
#12229=CARTESIAN_POINT ( 'NONE',  ( 22.85867476669663745, -36.41545538135959958, -16.50000000000000000 ) ) ;
#12233=DIRECTION ( 'NONE',  ( -0.000000000000000000, -0.000000000000000000, -1.000000000000000000 ) ) ;
#12239=CARTESIAN_POINT ( 'NONE',  ( 22.94541271838008356, -35.03073867843704647, -6.500000000000000888 ) ) ;
#12243=CARTESIAN_POINT ( 'NONE',  ( 32.74775157612609178, -27.21557300919356948, -19.50000000000000355 ) ) ;
#12247=CARTESIAN_POINT ( 'NONE',  ( 25.64627119138473432, -23.40052582045089480, -16.50000000000000000 ) ) ;
#12253=EDGE_CURVE ( 'NONE', #18281, #22584, #28073, .T. ) ;
#12264=AXIS2_PLACEMENT_3D ( 'NONE', #23038, #22897, #22738 ) ;
#12279=CYLINDRICAL_SURFACE ( 'NONE', #7922, 3.559164065751841743 ) ;
#12304=EDGE_LOOP ( 'NONE', ( #28467, #22760, #14006, #12954 ) ) ;
#12307=CARTESIAN_POINT ( 'NONE',  ( 32.24119435725080507, -26.76047165977712794, -16.50000600000000262 ) ) ;
#12328=DIRECTION ( 'NONE',  ( -0.000000000000000000, -0.000000000000000000, 1.000000000000000000 ) ) ;
#12346=CYLINDRICAL_SURFACE ( 'NONE', #1602, 3.559164065751841743 ) ;
#12358=CARTESIAN_POINT ( 'NONE',  ( -2.687479362164884034, -44.39187623478217404, -19.50000000000000355 ) ) ;
#12366=CARTESIAN_POINT ( 'NONE',  ( 37.98493438987956949, 11.12428508576150143, -1.500000000000000000 ) ) ;
#12383=DIRECTION ( 'NONE',  ( -0.000000000000000000, -0.000000000000000000, -1.000000000000000000 ) ) ;
#12394=CARTESIAN_POINT ( 'NONE',  ( 9.585801206154414444, -42.83572092346827276, -16.50000000000000355 ) ) ;
#12410=CYLINDRICAL_SURFACE ( 'NONE', #12458, 7.500000000000000000 ) ;
#12458=AXIS2_PLACEMENT_3D ( 'NONE', #16762, #229, #21746 ) ;
#12497=EDGE_LOOP ( 'NONE', ( #11110, #14403, #22918, #19652 ) ) ;
#12505=ORIENTED_EDGE ( 'NONE', *, *, #8876, .T. ) ;
#12518=CARTESIAN_POINT ( 'NONE',  ( -34.07766914599911701, 21.40380666528009002, -1.500000000000000000 ) ) ;
#12524=CARTESIAN_POINT ( 'NONE',  ( 31.18700685317022803, -26.11823559933272421, -1.500000000000000000 ) ) ;
#12581=CARTESIAN_POINT ( 'NONE',  ( -5.729465025513086419E-13, 44.07656359094158915, -16.50000000000000000 ) ) ;
#12583=VERTEX_POINT ( 'NONE', #18811 ) ;
#12605=AXIS2_PLACEMENT_3D ( 'NONE', #17600, #18220, #20092 ) ;
#12608=VECTOR ( 'NONE', #8182, 1000.000000000000000 ) ;
#12644=DIRECTION ( 'NONE',  ( -0.000000000000000000, -0.000000000000000000, -1.000000000000000000 ) ) ;
#12657=EDGE_CURVE ( 'NONE', #8571, #3296, #9406, .T. ) ;
#12682=CARTESIAN_POINT ( 'NONE',  ( 4.336808689942017736E-16, 42.50000000000000000, -1.500000000000000000 ) ) ;
#12688=CARTESIAN_POINT ( 'NONE',  ( -33.03678684150562361, -25.60268807474236752, -16.50000000000000000 ) ) ;
#12702=ORIENTED_EDGE ( 'NONE', *, *, #6331, .T. ) ;
#12711=CARTESIAN_POINT ( 'NONE',  ( -20.65888525914364493, -38.75220717792906555, -19.50000000000000355 ) ) ;
#12748=ORIENTED_EDGE ( 'NONE', *, *, #20311, .F. ) ;
#12749=ORIENTED_EDGE ( 'NONE', *, *, #18906, .T. ) ;
#12759=CARTESIAN_POINT ( 'NONE',  ( 40.57601884795947456, 0.2711064951079322771, -16.50000000000000000 ) ) ;
#12783=ADVANCED_FACE ( 'NONE', ( #5533 ), #12410, .F. ) ;
#12814=CARTESIAN_POINT ( 'NONE',  ( 22.58267429318970443, -26.57182937991349903, -6.499999999999999112 ) ) ;
#12817=EDGE_CURVE ( 'NONE', #30377, #29282, #5227, .T. ) ;
#12821=VECTOR ( 'NONE', #23169, 1000.000000000000000 ) ;
#12872=CARTESIAN_POINT ( 'NONE',  ( -32.74775157610760346, -27.21557300919352329, -19.50000000000000355 ) ) ;
#12878=CARTESIAN_POINT ( 'NONE',  ( -40.89187623478217404, -5.790488632116337797, -19.50000000000000355 ) ) ;
#12899=ORIENTED_EDGE ( 'NONE', *, *, #26014, .T. ) ;
#12905=FACE_OUTER_BOUND ( 'NONE', #1896, .T. ) ;
#12922=EDGE_LOOP ( 'NONE', ( #23429, #6936, #14762, #28139 ) ) ;
#12927=CARTESIAN_POINT ( 'NONE',  ( 40.53201937462365123, -2.366163742593401231, -16.50000000000000355 ) ) ;
#12928=ORIENTED_EDGE ( 'NONE', *, *, #22, .T. ) ;
#12944=PLANE ( 'NONE',  #23004 ) ;
#12954=ORIENTED_EDGE ( 'NONE', *, *, #22307, .T. ) ;
#12955=CARTESIAN_POINT ( 'NONE',  ( 20.71335220384823117, 27.86167394782616213, -6.500000000000000888 ) ) ;
#12973=EDGE_LOOP ( 'NONE', ( #24538, #9634 ) ) ;
#12992=CARTESIAN_POINT ( 'NONE',  ( 33.03677034811506275, 25.60271145924337688, -16.50000000000000000 ) ) ;
#13006=CARTESIAN_POINT ( 'NONE',  ( -23.27838112031802709, -36.10018649381529343, -16.50000600000000262 ) ) ;
#13011=CARTESIAN_POINT ( 'NONE',  ( 0.000000000000000000, 0.000000000000000000, -6.500000000000000888 ) ) ;
#13020=CARTESIAN_POINT ( 'NONE',  ( 13.22505861668094340, 42.10773672057246841, -19.50000000000000355 ) ) ;
#13026=CARTESIAN_POINT ( 'NONE',  ( -32.74775157610760346, -27.21557300919352329, -19.50000000000000355 ) ) ;
#13051=EDGE_CURVE ( 'NONE', #18178, #20109, #25432, .T. ) ;
#13053=CARTESIAN_POINT ( 'NONE',  ( -40.22788059446288145, 5.869150616580578905, -16.50000000000000000 ) ) ;
#13117=DIRECTION ( 'NONE',  ( 0.2972711322815261292, 0.9547931052914340189, 0.000000000000000000 ) ) ;
#13136=B_SPLINE_SURFACE_WITH_KNOTS ( 'NONE', 1, 3, ( 
 ( #11909, #30603, #6751, #14067, #2382, #18768, #6911, #23578, #2221, #41, #6604, #23898, #4874, #11289, #20783, #8957, #18472, #16121, #11447, #11739, #14688, #24191, #5497, #8001, #7835, #29045, #28899, #14998, #184, #24511, #12200, #19675, #2844, #10168, #19212, #26557, #24360, #3156, #17034, #17347, #19840, #12055 ),
 ( #12682, #9865, #22174, #802, #7687, #14846, #5336, #9703, #2690, #12366, #10324, #16886, #3006, #27025, #12524, #26873, #21548, #26706, #21700, #29196, #7534, #19379, #24040, #5185, #29363, #21869, #22017, #17505, #5653, #15148, #2541, #653, #28741, #19532, #7378, #26406, #342, #5030, #14544, #503, #10023, #17185 ) ),
 .UNSPECIFIED., .F., .T., .F.,
 ( 2, 2 ),
 ( 4, 2, 2, 2, 2, 2, 2, 2, 2, 2, 2, 2, 2, 2, 2, 2, 2, 2, 2, 2, 4 ),
 ( 0.000000000000000000, 1.000000000000000000 ),
 ( 0.000000000000000000, 0.1963495408493620697, 0.3926990816987241395, 0.7853981633974482790, 1.178097245096172418, 1.570796326794896558, 1.963495408493620697, 2.356194490192344837, 2.748893571891068976, 2.945243112740430824, 3.141592653589793116, 3.337942194439155408, 3.534291735288517255, 3.926990816987241395, 4.319689898685965090, 4.712388980384689674, 5.105088062083414258, 5.497787143782137953, 5.890486225480861648, 6.086835766330223940, 6.283185307179586232 ),
 .UNSPECIFIED. ) ;
#13147=DIRECTION ( 'NONE',  ( 1.000000000000000000, 0.000000000000000000, 0.000000000000000000 ) ) ;
#13164=DIRECTION ( 'NONE',  ( -0.000000000000000000, -0.000000000000000000, -1.000000000000000000 ) ) ;
#13170=ORIENTED_EDGE ( 'NONE', *, *, #22924, .T. ) ;
#13173=CARTESIAN_POINT ( 'NONE',  ( -34.07766914599908148, -21.40380666528021081, -1.500000000000000000 ) ) ;
#13175=B_SPLINE_CURVE_WITH_KNOTS ( 'NONE', 3,
 ( #28396, #7176, #2497, #26048, #16689, #26196, #4828, #14344, #23853, #22129 ),
 .UNSPECIFIED., .F., .F.,
 ( 4, 2, 2, 2, 4 ),
 ( 0.1536962897835600916, 0.3652722173376700687, 0.5768481448917800458, 0.7884240724458899674, 1.000000000000000000 ),
 .UNSPECIFIED. ) ;
#13180=CARTESIAN_POINT ( 'NONE',  ( 23.96732207937828463, 33.98584080152456011, -1.500000000000000000 ) ) ;
#13183=AXIS2_PLACEMENT_3D ( 'NONE', #1667, #18051, #3709 ) ;
#13192=EDGE_CURVE ( 'NONE', #544, #22552, #20872, .T. ) ;
#13214=CARTESIAN_POINT ( 'NONE',  ( -10.64374042650075403, -42.96126232887726815, -19.50000000000000355 ) ) ;
#13243=VECTOR ( 'NONE', #8242, 1000.000000000000000 ) ;
#13268=VERTEX_POINT ( 'NONE', #29517 ) ;
#13291=CARTESIAN_POINT ( 'NONE',  ( -24.03057240117691862, 26.57182937991349903, -6.500000000000000888 ) ) ;
#13305=ORIENTED_EDGE ( 'NONE', *, *, #17028, .T. ) ;
#13312=CARTESIAN_POINT ( 'NONE',  ( -22.94541271838176755, -35.03073867844241818, -6.500000000000000888 ) ) ;
#13326=CARTESIAN_POINT ( 'NONE',  ( -22.58267429318970443, -26.57182937991348481, -1.500000000000001332 ) ) ;
#13328=CARTESIAN_POINT ( 'NONE',  ( 32.74775157611827581, 27.21557300921217859, -19.50000000000000355 ) ) ;
#13334=CARTESIAN_POINT ( 'NONE',  ( 37.98493438987956949, 11.12428508576150143, -1.500000000000000000 ) ) ;
#13338=LINE ( 'NONE', #15507, #20378 ) ;
#13340=CARTESIAN_POINT ( 'NONE',  ( 37.98493438987956949, 11.12428508576150143, -1.500000000000000000 ) ) ;
#13350=AXIS2_PLACEMENT_3D ( 'NONE', #23791, #11791, #7119 ) ;
#13366=CARTESIAN_POINT ( 'NONE',  ( 32.82330813384209023, -22.94799032726822929, -1.500000000000000000 ) ) ;
#13373=CARTESIAN_POINT ( 'NONE',  ( -39.83602371821034183, 11.57901747687032490, -19.50000000000000355 ) ) ;
#13425=DIRECTION ( 'NONE',  ( -0.5503133621338232029, -0.8349582046168344540, 0.000000000000000000 ) ) ;
#13427=ORIENTED_EDGE ( 'NONE', *, *, #4084, .F. ) ;
#13438=CIRCLE ( 'NONE', #7949, 1.447898107987198646 ) ;
#13468=FACE_OUTER_BOUND ( 'NONE', #4369, .T. ) ;
#13493=CARTESIAN_POINT ( 'NONE',  ( 12.56641067637329812, 40.32935944495179115, -1.500000000000000000 ) ) ;
#13501=EDGE_CURVE ( 'NONE', #6837, #11031, #4079, .T. ) ;
#13512=ORIENTED_EDGE ( 'NONE', *, *, #8916, .F. ) ;
#13525=ORIENTED_EDGE ( 'NONE', *, *, #23837, .F. ) ;
#13528=CARTESIAN_POINT ( 'NONE',  ( 32.74775157612609178, -27.21557300919356948, -19.50000000000000355 ) ) ;
#13530=ORIENTED_EDGE ( 'NONE', *, *, #29982, .F. ) ;
#13540=CARTESIAN_POINT ( 'NONE',  ( -4.175048725057020960, -43.84342162469872051, -16.50000000000000355 ) ) ;
#13557=ORIENTED_EDGE ( 'NONE', *, *, #2658, .T. ) ;
#13575=DIRECTION ( 'NONE',  ( -0.000000000000000000, -0.000000000000000000, -1.000000000000000000 ) ) ;
#13583=ADVANCED_FACE ( 'NONE', ( #29910 ), #20531, .F. ) ;
#13585=EDGE_CURVE ( 'NONE', #6674, #21864, #6031, .T. ) ;
#13588=CARTESIAN_POINT ( 'NONE',  ( -40.05104235265675783, -2.353288714454540020, -6.500000000000000888 ) ) ;
#13593=ORIENTED_EDGE ( 'NONE', *, *, #4058, .T. ) ;
#13609=CARTESIAN_POINT ( 'NONE',  ( -26.80246859415415273, 7.028748154183637631, -1.499999999999999556 ) ) ;
#13626=VERTEX_POINT ( 'NONE', #25377 ) ;
#13651=CARTESIAN_POINT ( 'NONE',  ( -13.22505861668333083, 42.10773672057167261, -19.50000000000000355 ) ) ;
#13659=CIRCLE ( 'NONE', #19118, 1.447898107987198646 ) ;
#13676=VERTEX_POINT ( 'NONE', #25530 ) ;
#13680=CARTESIAN_POINT ( 'NONE',  ( 0.000000000000000000, 44.39187623478217404, -19.50000000000000355 ) ) ;
#13692=VERTEX_POINT ( 'NONE', #6193 ) ;
#13699=CARTESIAN_POINT ( 'NONE',  ( 8.321693349542481855, -43.14082846441630892, -16.50000000000000355 ) ) ;
#13717=DIRECTION ( 'NONE',  ( -1.000000000000000000, 0.000000000000000000, 0.000000000000000000 ) ) ;
#13756=CARTESIAN_POINT ( 'NONE',  ( -23.27838111883973227, 36.10018642694448943, -16.50000600000000262 ) ) ;
#13782=CARTESIAN_POINT ( 'NONE',  ( -26.80246859415415273, 7.028748154183637631, -1.499999999999999556 ) ) ;
#13791=VECTOR ( 'NONE', #13164, 1000.000000000000000 ) ;
#13792=CARTESIAN_POINT ( 'NONE',  ( 10.11202017158463917, -41.14070756921186955, -1.500000000000000000 ) ) ;
#13796=CARTESIAN_POINT ( 'NONE',  ( -25.23756106473024730, -11.43858098102957577, -16.50000000000000000 ) ) ;
#13808=DIRECTION ( 'NONE',  ( 0.2972711322815266843, -0.9547931052914339078, 0.000000000000000000 ) ) ;
#13819=DIRECTION ( 'NONE',  ( 0.000000000000000000, 0.000000000000000000, 1.000000000000000000 ) ) ;
#13825=CARTESIAN_POINT ( 'NONE',  ( 12.56641067637329812, 40.32935944495179115, -1.500000000000000000 ) ) ;
#13839=CARTESIAN_POINT ( 'NONE',  ( -14.49834914336386404, -41.18788872621845343, -16.50000000000000355 ) ) ;
#13848=CARTESIAN_POINT ( 'NONE',  ( -39.87350638641186862, -4.706224724276806270, -11.49999999999999645 ) ) ;
#13853=DIRECTION ( 'NONE',  ( -0.2972711322815276280, -0.9547931052914334638, 0.000000000000000000 ) ) ;
#13856=EDGE_LOOP ( 'NONE', ( #22548, #5122, #20528, #7220 ) ) ;
#13860=AXIS2_PLACEMENT_3D ( 'NONE', #27277, #5910, #20700 ) ;
#13883=CARTESIAN_POINT ( 'NONE',  ( 20.55390841643019684, -27.45161667029107022, -16.50001200000000168 ) ) ;
#13909=EDGE_CURVE ( 'NONE', #22584, #26952, #13338, .T. ) ;
#13911=CARTESIAN_POINT ( 'NONE',  ( -23.07229726322976404, 36.25693017875646262, -16.50000000000000000 ) ) ;
#13924=CARTESIAN_POINT ( 'NONE',  ( 25.19442432474404470, 35.44676296256560022, -19.50000000000000355 ) ) ;
#13938=VERTEX_POINT ( 'NONE', #30164 ) ;
#13945=CARTESIAN_POINT ( 'NONE',  ( -32.93066664481271033, 23.11087910253402455, -3.166603179814979185 ) ) ;
#13970=VERTEX_POINT ( 'NONE', #14077 ) ;
#13972=CARTESIAN_POINT ( 'NONE',  ( 37.98493438987956949, 11.12428508576150143, -1.500000000000000000 ) ) ;
#13983=EDGE_CURVE ( 'NONE', #5019, #7694, #26091, .T. ) ;
#13995=CARTESIAN_POINT ( 'NONE',  ( 7.295277785476350196, -43.36226450306268987, -16.50000000000000000 ) ) ;
#14001=VERTEX_POINT ( 'NONE', #16276 ) ;
#14006=ORIENTED_EDGE ( 'NONE', *, *, #23471, .T. ) ;
#14010=VECTOR ( 'NONE', #17456, 1000.000000000000114 ) ;
#14018=CARTESIAN_POINT ( 'NONE',  ( -31.29501345865439532, 26.27841684421964885, -6.500000000000000888 ) ) ;
#14020=ORIENTED_EDGE ( 'NONE', *, *, #27092, .F. ) ;
#14029=LINE ( 'NONE', #14335, #23199 ) ;
#14030=DIRECTION ( 'NONE',  ( 0.000000000000000000, -0.000000000000000000, 1.000000000000000000 ) ) ;
#14038=DIRECTION ( 'NONE',  ( 0.06975647374412530244, -0.000000000000000000, 0.9975640502598241977 ) ) ;
#14052=CARTESIAN_POINT ( 'NONE',  ( -40.05104235265675783, 2.353288714454549790, -11.49999999999999645 ) ) ;
#14060=CARTESIAN_POINT ( 'NONE',  ( 32.74775157611827581, 27.21557300921217859, -19.50000000000000355 ) ) ;
#14065=CARTESIAN_POINT ( 'NONE',  ( -33.53985793123796100, 24.80925987296827984, -16.50000000000000000 ) ) ;
#14067=CARTESIAN_POINT ( 'NONE',  ( 10.64374042650142904, 42.96126232887663576, -19.50000000000000355 ) ) ;
#14070=CIRCLE ( 'NONE', #15576, 1.447898107987198646 ) ;
#14072=CARTESIAN_POINT ( 'NONE',  ( -34.07766914599911701, 21.40380666528009002, -1.500000000000000000 ) ) ;
#14077=CARTESIAN_POINT ( 'NONE',  ( 20.47140833542507821, -26.57182937991349903, -6.500000000000000888 ) ) ;
#14078=CARTESIAN_POINT ( 'NONE',  ( 19.64114023396309960, -37.13592150529014191, -1.500000000000000000 ) ) ;
#14088=VERTEX_POINT ( 'NONE', #23437 ) ;
#14104=CARTESIAN_POINT ( 'NONE',  ( 31.31394823341868161, -25.51108937476379879, -1.500000000000000000 ) ) ;
#14108=CARTESIAN_POINT ( 'NONE',  ( 0.000000000000000000, 44.39187623478217404, -19.50000000000000355 ) ) ;
#14109=LINE ( 'NONE', #23617, #18869 ) ;
#14130=CARTESIAN_POINT ( 'NONE',  ( 26.80246859415415273, 7.028748154183637631, -6.500000000000000888 ) ) ;
#14134=CARTESIAN_POINT ( 'NONE',  ( 16.18102710830015667, -40.48237095587791856, -16.50000000000000355 ) ) ;
#14155=ORIENTED_EDGE ( 'NONE', *, *, #25631, .T. ) ;
#14166=EDGE_CURVE ( 'NONE', #5019, #2261, #18677, .T. ) ;
#14184=LINE ( 'NONE', #25741, #2900 ) ;
#14189=ORIENTED_EDGE ( 'NONE', *, *, #22201, .T. ) ;
#14192=LINE ( 'NONE', #9378, #6980 ) ;
#14198=UNCERTAINTY_MEASURE_WITH_UNIT (LENGTH_MEASURE( 1.000000000000000082E-05 ), #29664, 'distance_accuracy_value', 'NONE');
#14209=CARTESIAN_POINT ( 'NONE',  ( -39.83602371821029919, -11.57901747687044924, -19.50000000000000355 ) ) ;
#14211=CARTESIAN_POINT ( 'NONE',  ( 25.47847050916411504, 26.57182937991349903, 26.54355021145563143 ) ) ;
#14221=DIRECTION ( 'NONE',  ( -0.000000000000000000, -0.000000000000000000, -1.000000000000000000 ) ) ;
#14240=CARTESIAN_POINT ( 'NONE',  ( 0.000000000000000000, 0.000000000000000000, -1.500000000000000000 ) ) ;
#14255=CARTESIAN_POINT ( 'NONE',  ( 33.46566279634969021, 23.92259740141769342, -11.49999999999999822 ) ) ;
#14257=CARTESIAN_POINT ( 'NONE',  ( -37.98493438988128901, 11.12428508575241004, -1.500000000000000000 ) ) ;
#14277=CARTESIAN_POINT ( 'NONE',  ( -31.31394823341925715, -25.51108937476197980, -1.500000000000000000 ) ) ;
#14291=ORIENTED_EDGE ( 'NONE', *, *, #28016, .F. ) ;
#14314=ORIENTED_EDGE ( 'NONE', *, *, #29046, .T. ) ;
#14324=DIRECTION ( 'NONE',  ( -0.2972711322815276280, -0.9547931052914334638, 0.000000000000000000 ) ) ;
#14330=ADVANCED_FACE ( 'NONE', ( #13468 ), #27182, .F. ) ;
#14333=CARTESIAN_POINT ( 'NONE',  ( 4.770489558936219510E-15, -42.50000000000000000, -1.500000000000000000 ) ) ;
#14335=CARTESIAN_POINT ( 'NONE',  ( 39.52380524533145945, -7.028748154382054913, -1.499999999999999556 ) ) ;
#14344=CARTESIAN_POINT ( 'NONE',  ( 24.49591551883469265, -22.99161772365830814, -16.50001200000000523 ) ) ;
#14347=CARTESIAN_POINT ( 'NONE',  ( 0.000000000000000000, 0.000000000000000000, -11.49999999999999645 ) ) ;
#14351=( GEOMETRIC_REPRESENTATION_CONTEXT ( 3 ) GLOBAL_UNCERTAINTY_ASSIGNED_CONTEXT ( ( #17008 ) ) GLOBAL_UNIT_ASSIGNED_CONTEXT ( ( #9640, #2297, #4337 ) ) REPRESENTATION_CONTEXT ( 'NONE', 'WORKASPACE' ) );
#14363=VERTEX_POINT ( 'NONE', #18580 ) ;
#14367=CARTESIAN_POINT ( 'NONE',  ( -4.183878327245746931, 43.84516588455117869, -16.50000000000000000 ) ) ;
#14374=CARTESIAN_POINT ( 'NONE',  ( -29.15452456067357545, -29.11038375075818152, -6.500000000000000888 ) ) ;
#14381=CARTESIAN_POINT ( 'NONE',  ( 31.18700685317022803, -26.11823559933272421, -1.500000000000000000 ) ) ;
#14382=DIRECTION ( 'NONE',  ( -0.000000000000000000, -0.000000000000000000, -1.000000000000000000 ) ) ;
#14400=B_SPLINE_CURVE_WITH_KNOTS ( 'NONE', 3,
 ( #8091, #17595, #27113, #15228, #24757, #8704 ),
 .UNSPECIFIED., .F., .F.,
 ( 4, 2, 4 ),
 ( 1.408367944307646891, 1.570796326794821507, 1.733224709277370712 ),
 .UNSPECIFIED. ) ;
#14403=ORIENTED_EDGE ( 'NONE', *, *, #27123, .T. ) ;
#14428=CARTESIAN_POINT ( 'NONE',  ( 4.770489558936219510E-15, -42.50000000000000000, -1.500000000000000000 ) ) ;
#14433=CARTESIAN_POINT ( 'NONE',  ( 25.64627119138473432, 23.40052582045089480, -16.50000000000000000 ) ) ;
#14451=CARTESIAN_POINT ( 'NONE',  ( 12.04446003218043515, 42.09125592553625239, -16.50000000000000000 ) ) ;
#14481=CARTESIAN_POINT ( 'NONE',  ( 31.29501345865701012, -26.27841684422097401, -6.499999999999999112 ) ) ;
#14500=CARTESIAN_POINT ( 'NONE',  ( 39.87350638640861433, 4.706224724276823146, -11.49999999999999645 ) ) ;
#14503=CARTESIAN_POINT ( 'NONE',  ( -40.05104235265675783, -2.353288714459718989, -11.49999999999999645 ) ) ;
#14520=CARTESIAN_POINT ( 'NONE',  ( -33.03787114093149313, 23.27353420009350415, -4.833239141675061745 ) ) ;
#14522=EDGE_LOOP ( 'NONE', ( #16996, #9191, #6467, #21058 ) ) ;
#14525=DIRECTION ( 'NONE',  ( -0.06975647374412530244, 0.000000000000000000, 0.9975640502598241977 ) ) ;
#14534=CARTESIAN_POINT ( 'NONE',  ( -31.18700685316100163, -26.11823559932341610, -1.500000000000000000 ) ) ;
#14535=DIRECTION ( 'NONE',  ( 0.000000000000000000, 0.000000000000000000, -1.000000000000000000 ) ) ;
#14536=EDGE_CURVE ( 'NONE', #28753, #16453, #2009, .T. ) ;
#14544=CARTESIAN_POINT ( 'NONE',  ( -10.11202017158466759, 41.14070756921185534, -1.500000000000000000 ) ) ;
#14549=EDGE_CURVE ( 'NONE', #7038, #23836, #13175, .T. ) ;
#14560=ORIENTED_EDGE ( 'NONE', *, *, #9154, .T. ) ;
#14580=FACE_OUTER_BOUND ( 'NONE', #10173, .T. ) ;
#14604=LINE ( 'NONE', #5404, #23774 ) ;
#14608=VECTOR ( 'NONE', #23585, 1000.000000000000114 ) ;
#14614=FACE_BOUND ( 'NONE', #24850, .T. ) ;
#14620=EDGE_LOOP ( 'NONE', ( #22438, #20944, #28134, #4208 ) ) ;
#14625=SHAPE_REPRESENTATION_RELATIONSHIP ( 'NONE' , 'NONE' ,  #16871, #8388 ) ;
#14649=VERTEX_POINT ( 'NONE', #14962 ) ;
#14651=DIRECTION ( 'NONE',  ( -0.8910248307962438385, 0.4539545692076743522, 0.000000000000000000 ) ) ;
#14658=ORIENTED_EDGE ( 'NONE', *, *, #14166, .T. ) ;
#14677=ORIENTED_EDGE ( 'NONE', *, *, #13983, .T. ) ;
#14680=CARTESIAN_POINT ( 'NONE',  ( 2.687479362164894248, -44.39187623478217404, -19.50000000000000355 ) ) ;
#14688=CARTESIAN_POINT ( 'NONE',  ( 2.687479362164894248, -44.39187623478217404, -19.50000000000000355 ) ) ;
#14706=LINE ( 'NONE', #29218, #19267 ) ;
#14709=CARTESIAN_POINT ( 'NONE',  ( 40.05520465696179855, -7.028746455191999587, -16.50000000000000000 ) ) ;
#14710=CARTESIAN_POINT ( 'NONE',  ( -21.90865045291187485, 23.69204963285887899, -16.50001200000000523 ) ) ;
#14714=CARTESIAN_POINT ( 'NONE',  ( 4.186421491866439304, -43.85598367614507964, -16.50000000000000000 ) ) ;
#14730=LINE ( 'NONE', #12247, #20605 ) ;
#14731=VERTEX_POINT ( 'NONE', #20706 ) ;
#14747=EDGE_LOOP ( 'NONE', ( #9845, #14020, #13557, #16355 ) ) ;
#14750=FACE_BOUND ( 'NONE', #12180, .T. ) ;
#14751=B_SPLINE_CURVE_WITH_KNOTS ( 'NONE', 3,
 ( #9390, #12039, #21534, #18747, #169 ),
 .UNSPECIFIED., .F., .F.,
 ( 4, 1, 4 ),
 ( 0.8465381644365373992, 0.8518173996194324804, 0.8570966348023274506 ),
 .UNSPECIFIED. ) ;
#14757=( GEOMETRIC_REPRESENTATION_CONTEXT ( 3 ) GLOBAL_UNCERTAINTY_ASSIGNED_CONTEXT ( ( #14198 ) ) GLOBAL_UNIT_ASSIGNED_CONTEXT ( ( #29664, #27485, #22631 ) ) REPRESENTATION_CONTEXT ( 'NONE', 'WORKASPACE' ) );
#14762=ORIENTED_EDGE ( 'NONE', *, *, #21005, .T. ) ;
#14777=B_SPLINE_CURVE_WITH_KNOTS ( 'NONE', 3,
 ( #26428, #5057, #16745, #7233, #5211, #26108, #28611 ),
 .UNSPECIFIED., .F., .F.,
 ( 4, 3, 4 ),
 ( 0.000000000000000000, 0.005031266826504186655, 0.01006253384358471795 ),
 .UNSPECIFIED. ) ;
#14808=CIRCLE ( 'NONE', #25769, 27.70876437800068359 ) ;
#14828=DIRECTION ( 'NONE',  ( 0.000000000000000000, 0.000000000000000000, -1.000000000000000000 ) ) ;
#14838=CARTESIAN_POINT ( 'NONE',  ( -35.76344986165608475, 22.29344514668535027, -19.50000000000000355 ) ) ;
#14846=CARTESIAN_POINT ( 'NONE',  ( 19.64114023396890829, 37.13592150528549496, -1.500000000000000000 ) ) ;
#14852=EDGE_LOOP ( 'NONE', ( #16816, #2645 ) ) ;
#14857=ORIENTED_EDGE ( 'NONE', *, *, #17035, .T. ) ;
#14862=ORIENTED_EDGE ( 'NONE', *, *, #19457, .T. ) ;
#14877=VECTOR ( 'NONE', #17724, 1000.000000000000000 ) ;
#14899=ORIENTED_EDGE ( 'NONE', *, *, #26128, .T. ) ;
#14932=ORIENTED_EDGE ( 'NONE', *, *, #5573, .F. ) ;
#14937=ORIENTED_EDGE ( 'NONE', *, *, #13909, .F. ) ;
#14962=CARTESIAN_POINT ( 'NONE',  ( 22.58267429318971864, 26.57182937991349903, -1.500000000000001332 ) ) ;
#14984=CIRCLE ( 'NONE', #23953, 3.559164065751841743 ) ;
#14989=ORIENTED_EDGE ( 'NONE', *, *, #19853, .T. ) ;
#14998=CARTESIAN_POINT ( 'NONE',  ( -32.74775157610760346, -27.21557300919352329, -19.50000000000000355 ) ) ;
#15005=CARTESIAN_POINT ( 'NONE',  ( -32.51029891075602052, -26.37762732681785494, -16.50000000000000000 ) ) ;
#15029=CARTESIAN_POINT ( 'NONE',  ( 4.336808689942017736E-16, 42.50000000000000000, -1.500000000000000000 ) ) ;
#15048=ORIENTED_EDGE ( 'NONE', *, *, #7357, .F. ) ;
#15053=VERTEX_POINT ( 'NONE', #571 ) ;
#15080=CARTESIAN_POINT ( 'NONE',  ( 40.57596378766727696, -1.195117231327979868, -16.50000000000000000 ) ) ;
#15091=CARTESIAN_POINT ( 'NONE',  ( 31.92585768990164397, -26.59981599195955226, -13.16665969525543289 ) ) ;
#15115=CARTESIAN_POINT ( 'NONE',  ( -31.76816150326424548, -26.51947378151102086, -11.49999299637583228 ) ) ;
#15116=EDGE_CURVE ( 'NONE', #20109, #18178, #13659, .T. ) ;
#15148=CARTESIAN_POINT ( 'NONE',  ( -37.98493438988125348, -11.12428508575252728, -1.500000000000000000 ) ) ;
#15157=PLANE ( 'NONE',  #3517 ) ;
#15158=ORIENTED_EDGE ( 'NONE', *, *, #20072, .T. ) ;
#15179=ORIENTED_EDGE ( 'NONE', *, *, #24286, .F. ) ;
#15182=CARTESIAN_POINT ( 'NONE',  ( -2.687479362164884034, -44.39187623478217404, -19.50000000000000355 ) ) ;
#15184=CARTESIAN_POINT ( 'NONE',  ( 25.23756106473024730, -11.43858098102957399, -16.50000000000000000 ) ) ;
#15185=ORIENTED_EDGE ( 'NONE', *, *, #6336, .F. ) ;
#15195=LINE ( 'NONE', #24721, #27791 ) ;
#15207=VERTEX_POINT ( 'NONE', #4002 ) ;
#15217=LINE ( 'NONE', #26958, #25627 ) ;
#15218=AXIS2_PLACEMENT_3D ( 'NONE', #22066, #10218, #19728 ) ;
#15221=ADVANCED_FACE ( 'NONE', ( #1051 ), #27069, .T. ) ;
#15222=DIRECTION ( 'NONE',  ( 0.8910248307962438385, 0.4539545692076743522, 0.000000000000000000 ) ) ;
#15226=ORIENTED_EDGE ( 'NONE', *, *, #19478, .F. ) ;
#15228=CARTESIAN_POINT ( 'NONE',  ( 40.05104235265675783, 2.353288714454550679, -11.49999999999999645 ) ) ;
#15260=CARTESIAN_POINT ( 'NONE',  ( -31.61046531695933837, -26.43913157123191482, -9.833326300989435609 ) ) ;
#15303=ADVANCED_FACE ( 'NONE', ( #19718 ), #28088, .T. ) ;
#15339=CARTESIAN_POINT ( 'NONE',  ( -10.64374042650075403, -42.96126232887726815, -19.50000000000000355 ) ) ;
#15342=ORIENTED_EDGE ( 'NONE', *, *, #6695, .T. ) ;
#15346=CARTESIAN_POINT ( 'NONE',  ( 19.64114023396309960, -37.13592150529014191, -1.500000000000000000 ) ) ;
#15350=CARTESIAN_POINT ( 'NONE',  ( 35.76344986165623396, 22.29344514668041199, -19.50000000000000355 ) ) ;
#15368=ADVANCED_FACE ( 'NONE', ( #15972 ), #20787, .F. ) ;
#15369=CARTESIAN_POINT ( 'NONE',  ( -40.35775004261427767, 4.707207311767386493, -16.50000000000000711 ) ) ;
#15383=CARTESIAN_POINT ( 'NONE',  ( 13.22505861668195237, -42.10773672056998862, -19.50000000000000355 ) ) ;
#15411=DIRECTION ( 'NONE',  ( -0.000000000000000000, -0.000000000000000000, -1.000000000000000000 ) ) ;
#15415=CARTESIAN_POINT ( 'NONE',  ( 25.64627119138473432, -23.40052582045089480, -16.50001200000000168 ) ) ;
#15460=CARTESIAN_POINT ( 'NONE',  ( -20.71335220384823117, -27.86167394782616213, -6.500000000000000888 ) ) ;
#15461=CARTESIAN_POINT ( 'NONE',  ( -40.05520497409654013, 7.028746409781321702, -16.50000000000000000 ) ) ;
#15472=ORIENTED_EDGE ( 'NONE', *, *, #11025, .F. ) ;
#15474=VECTOR ( 'NONE', #16199, 1000.000000000000000 ) ;
#15484=CYLINDRICAL_SURFACE ( 'NONE', #18815, 1.447898107987198646 ) ;
#15497=CARTESIAN_POINT ( 'NONE',  ( 32.74775157612609178, -27.21557300919356948, -19.50000000000000355 ) ) ;
#15503=CARTESIAN_POINT ( 'NONE',  ( 10.64374042650304020, -42.96126232887725394, -19.50000000000000355 ) ) ;
#15505=DIRECTION ( 'NONE',  ( -1.000000000000000000, 0.000000000000000000, 0.000000000000000000 ) ) ;
#15507=CARTESIAN_POINT ( 'NONE',  ( -20.71335220384823117, 27.86167394782616213, -6.500000000000000888 ) ) ;
#15508=CARTESIAN_POINT ( 'NONE',  ( 4.336808689942017736E-16, 42.50000000000000000, -1.500000000000000000 ) ) ;
#15576=AXIS2_PLACEMENT_3D ( 'NONE', #1484, #8348, #15505 ) ;
#15577=AXIS2_PLACEMENT_3D ( 'NONE', #11999, #21491, #6696 ) ;
#15610=ORIENTED_EDGE ( 'NONE', *, *, #17204, .T. ) ;
#15620=CARTESIAN_POINT ( 'NONE',  ( -24.03057240117690441, -26.57182937991348481, -6.499999999999999112 ) ) ;
#15634=PLANE ( 'NONE',  #5827 ) ;
#15640=DIRECTION ( 'NONE',  ( -0.2972711322815276280, -0.9547931052914334638, 0.000000000000000000 ) ) ;
#15646=CARTESIAN_POINT ( 'NONE',  ( 33.16313691975489064, 0.000000000000000000, -1.500000000000000000 ) ) ;
#15653=CARTESIAN_POINT ( 'NONE',  ( -20.65888525914364493, -38.75220717792906555, -19.50000000000000355 ) ) ;
#15658=ORIENTED_EDGE ( 'NONE', *, *, #17908, .F. ) ;
#15659=CARTESIAN_POINT ( 'NONE',  ( 34.07766914600081520, 21.40380666527109810, -1.500000000000000000 ) ) ;
#15674=EDGE_CURVE ( 'NONE', #22154, #18657, #27605, .T. ) ;
#15704=ORIENTED_EDGE ( 'NONE', *, *, #14166, .F. ) ;
#15753=ORIENTED_EDGE ( 'NONE', *, *, #22707, .F. ) ;
#15785=B_SPLINE_CURVE_WITH_KNOTS ( 'NONE', 1,
 ( #23677, #14333 ),
 .UNSPECIFIED., .F., .F.,
 ( 2, 2 ),
 ( 0.1666666666666656582, 1.000000000000000000 ),
 .UNSPECIFIED. ) ;
#15788=CARTESIAN_POINT ( 'NONE',  ( -23.05654803992426949, -35.38768971485402659, -9.833278432273298009 ) ) ;
#15806=CARTESIAN_POINT ( 'NONE',  ( -23.96732207939035675, 33.98584080153585774, -1.500000000000000000 ) ) ;
#15809=CIRCLE ( 'NONE', #27779, 1.447898107987198646 ) ;
#15812=CARTESIAN_POINT ( 'NONE',  ( 31.18700685317022803, -26.11823559933272421, -1.500000000000000000 ) ) ;
#15819=CARTESIAN_POINT ( 'NONE',  ( 20.65888525914559892, 38.75220717792412728, -19.50000000000000355 ) ) ;
#15843=DIRECTION ( 'NONE',  ( -1.000000000000000000, 0.000000000000000000, 0.000000000000000000 ) ) ;
#15852=CARTESIAN_POINT ( 'NONE',  ( 5.374868878255610660, 44.10336124695606230, -19.50000000000000355 ) ) ;
#15867=VECTOR ( 'NONE', #12383, 1000.000000000000000 ) ;
#15868=CARTESIAN_POINT ( 'NONE',  ( -2.350907959953084880, -44.02170661032951671, -16.49999999999999645 ) ) ;
#15872=VERTEX_POINT ( 'NONE', #23973 ) ;
#15876=CARTESIAN_POINT ( 'NONE',  ( -39.70095622563229654, 7.028748154183642072, -13.16666434799648755 ) ) ;
#15898=ORIENTED_EDGE ( 'NONE', *, *, #2912, .F. ) ;
#15915=EDGE_CURVE ( 'NONE', #19456, #28062, #15217, .T. ) ;
#15956=DIRECTION ( 'NONE',  ( -0.5503133621338236470, 0.8349582046168341209, 0.000000000000000000 ) ) ;
#15968=CARTESIAN_POINT ( 'NONE',  ( 5.105024945673418912, -42.22604126506271882, -1.500000000000000000 ) ) ;
#15972=FACE_OUTER_BOUND ( 'NONE', #9487, .T. ) ;
#15978=CARTESIAN_POINT ( 'NONE',  ( 35.76344986163714168, -22.29344514668044752, -19.50000000000000355 ) ) ;
#15982=ADVANCED_FACE ( 'NONE', ( #21797 ), #30361, .F. ) ;
#15999=DIRECTION ( 'NONE',  ( -0.8910248307962436165, -0.4539545692076746852, 0.000000000000000000 ) ) ;
#16002=CARTESIAN_POINT ( 'NONE',  ( 0.000000000000000000, 0.000000000000000000, -16.50000000000000000 ) ) ;
#16003=ORIENTED_EDGE ( 'NONE', *, *, #4185, .F. ) ;
#16006=CARTESIAN_POINT ( 'NONE',  ( -13.22505861668184046, -42.10773672057003125, -19.50000000000000355 ) ) ;
#16060=PRODUCT_DEFINITION_CONTEXT ( 'detailed design', #5010, 'design' ) ;
#16080=DIRECTION ( 'NONE',  ( -1.000000000000000000, -9.769962616701377556E-15, 0.000000000000000000 ) ) ;
#16098=VERTEX_POINT ( 'NONE', #26608 ) ;
#16101=CARTESIAN_POINT ( 'NONE',  ( -1.832066046471847676, 44.03802034382739805, -16.49999999999999645 ) ) ;
#16106=CARTESIAN_POINT ( 'NONE',  ( -25.32744450373244050, -23.23809170341762353, -16.50001200000000168 ) ) ;
#16119=CARTESIAN_POINT ( 'NONE',  ( 2.552544030762014415, -42.50000000000000000, -1.500000000000000000 ) ) ;
#16121=CARTESIAN_POINT ( 'NONE',  ( 13.22505861668195237, -42.10773672056998862, -19.50000000000000355 ) ) ;
#16156=VERTEX_POINT ( 'NONE', #29411 ) ;
#16199=DIRECTION ( 'NONE',  ( 1.000000000000000000, -0.000000000000000000, 0.000000000000000000 ) ) ;
#16206=CARTESIAN_POINT ( 'NONE',  ( -20.71335220384823117, -27.86167394782616213, -6.500000000000000888 ) ) ;
#16242=CARTESIAN_POINT ( 'NONE',  ( -21.80735578196799196, 37.17533440937560840, -16.50000000000000000 ) ) ;
#16256=FACE_OUTER_BOUND ( 'NONE', #27684, .T. ) ;
#16265=CARTESIAN_POINT ( 'NONE',  ( -39.00000000000000000, 5.563236990218665134, -1.500000000000000000 ) ) ;
#16270=CARTESIAN_POINT ( 'NONE',  ( 4.336808689942017736E-16, 42.50000000000000000, -1.500000000000000000 ) ) ;
#16272=ADVANCED_FACE ( 'NONE', ( #1322 ), #17343, .T. ) ;
#16276=CARTESIAN_POINT ( 'NONE',  ( 20.71335220384823117, -27.86167394782616213, -6.500000000000000888 ) ) ;
#16278=CARTESIAN_POINT ( 'NONE',  ( -5.105024945673440229, 42.22604126506271172, -1.500000000000000000 ) ) ;
#16301=CARTESIAN_POINT ( 'NONE',  ( 24.03057240117691862, -26.57182937991349903, -6.500000000000000888 ) ) ;
#16309=VECTOR ( 'NONE', #25573, 1000.000000000000000 ) ;
#16326=CARTESIAN_POINT ( 'NONE',  ( -15.69194956178364109, -40.64901747633663831, -16.49999999999999645 ) ) ;
#16328=VERTEX_POINT ( 'NONE', #11298 ) ;
#16355=ORIENTED_EDGE ( 'NONE', *, *, #27689, .T. ) ;
#16361=PLANE ( 'NONE',  #8518 ) ;
#16363=ORIENTED_EDGE ( 'NONE', *, *, #20994, .T. ) ;
#16365=CIRCLE ( 'NONE', #17346, 1.447898107987198646 ) ;
#16385=CIRCLE ( 'NONE', #23859, 3.559164065751841743 ) ;
#16434=EDGE_CURVE ( 'NONE', #24153, #18657, #1574, .T. ) ;
#16453=VERTEX_POINT ( 'NONE', #7697 ) ;
#16473=VERTEX_POINT ( 'NONE', #12064 ) ;
#16480=CARTESIAN_POINT ( 'NONE',  ( 0.000000000000000000, 0.000000000000000000, -11.49999999999999645 ) ) ;
#16489=CARTESIAN_POINT ( 'NONE',  ( 23.27838111857050407, -36.10018641471199174, -16.50000599999999906 ) ) ;
#16492=CARTESIAN_POINT ( 'NONE',  ( 1.734723475976807094E-15, 44.07656352898514740, -6.500000000000000888 ) ) ;
#16515=DIRECTION ( 'NONE',  ( -1.000000000000000000, 0.000000000000000000, 0.000000000000000000 ) ) ;
#16523=DIRECTION ( 'NONE',  ( -0.000000000000000000, -0.000000000000000000, -1.000000000000000000 ) ) ;
#16530=CARTESIAN_POINT ( 'NONE',  ( -29.55332031600174858, 27.89853503084644260, -1.500000000000009992 ) ) ;
#16531=CARTESIAN_POINT ( 'NONE',  ( -39.52380524535560369, 7.028748154183623420, -11.49999999999999645 ) ) ;
#16557=CARTESIAN_POINT ( 'NONE',  ( 39.00000000000000000, -5.563236990218592304, -1.500000000000000000 ) ) ;
#16558=LINE ( 'NONE', #14211, #20760 ) ;
#16578=CARTESIAN_POINT ( 'NONE',  ( -31.18700685316050780, 26.11823559932051353, -1.500000000000000000 ) ) ;
#16579=LINE ( 'NONE', #26716, #6003 ) ;
#16581=EDGE_LOOP ( 'NONE', ( #27940, #6860 ) ) ;
#16592=CARTESIAN_POINT ( 'NONE',  ( 32.82330813384650270, 22.94799032727486932, -1.500000000000000000 ) ) ;
#16610=ORIENTED_EDGE ( 'NONE', *, *, #28026, .F. ) ;
#16611=ORIENTED_EDGE ( 'NONE', *, *, #29046, .F. ) ;
#16614=CARTESIAN_POINT ( 'NONE',  ( -23.96732207938974213, -33.98584080153308662, -1.500000000000000000 ) ) ;
#16636=B_SPLINE_CURVE_WITH_KNOTS ( 'NONE', 3,
 ( #18027, #11005, #20803, #30329, #18179, #18486, #6623 ),
 .UNSPECIFIED., .F., .F.,
 ( 4, 3, 4 ),
 ( 0.000000000000000000, 0.005028111721571001773, 0.01005622344661834602 ),
 .UNSPECIFIED. ) ;
#16637=B_SPLINE_CURVE_WITH_KNOTS ( 'NONE', 3,
 ( #1630, #17687, #11141, #29697, #6295, #20339, #27666 ),
 .UNSPECIFIED., .F., .F.,
 ( 4, 3, 4 ),
 ( 0.000000000000000000, 0.005031266823721201875, 0.01006253384080261354 ),
 .UNSPECIFIED. ) ;
#16639=CARTESIAN_POINT ( 'NONE',  ( -32.82330813384598400, -22.94799032726886523, -1.500000000000000000 ) ) ;
#16643=CARTESIAN_POINT ( 'NONE',  ( -32.81350286003733885, 7.028748154183637631, -6.500000000000000888 ) ) ;
#16646=DIRECTION ( 'NONE',  ( -0.000000000000000000, -0.000000000000000000, 1.000000000000000000 ) ) ;
#16647=FACE_OUTER_BOUND ( 'NONE', #23830, .T. ) ;
#16650=EDGE_LOOP ( 'NONE', ( #29810, #25928, #16363, #27660 ) ) ;
#16671=ORIENTED_EDGE ( 'NONE', *, *, #28234, .F. ) ;
#16688=FACE_OUTER_BOUND ( 'NONE', #7997, .T. ) ;
#16689=CARTESIAN_POINT ( 'NONE',  ( 21.65446070919043109, -23.85364010248227018, -16.50001200000000168 ) ) ;
#16704=CARTESIAN_POINT ( 'NONE',  ( -16.18009747266616571, 40.48382543897108832, -16.50000000000000355 ) ) ;
#16707=CARTESIAN_POINT ( 'NONE',  ( -39.87350638641265732, -4.706224724266461656, -11.49999999999999645 ) ) ;
#16716=CARTESIAN_POINT ( 'NONE',  ( 5.105024945674004222, 42.22604126506330857, -1.500000000000000000 ) ) ;
#16720=DIRECTION ( 'NONE',  ( 0.8910248307962433945, -0.4539545692076750738, 0.000000000000000000 ) ) ;
#16743=LINE ( 'NONE', #23599, #4325 ) ;
#16745=CARTESIAN_POINT ( 'NONE',  ( 23.16753610420047949, 35.74416778161837982, -13.16661230991478071 ) ) ;
#16758=CARTESIAN_POINT ( 'NONE',  ( 23.96732207938043402, -33.98584080152387088, -1.500000000000000000 ) ) ;
#16761=ORIENTED_EDGE ( 'NONE', *, *, #30561, .F. ) ;
#16762=CARTESIAN_POINT ( 'NONE',  ( 0.000000000000000000, 0.000000000000000000, 63.50000000000000000 ) ) ;
#16784=DIRECTION ( 'NONE',  ( -0.000000000000000000, -0.000000000000000000, -1.000000000000000000 ) ) ;
#16787=ORIENTED_EDGE ( 'NONE', *, *, #25211, .T. ) ;
#16796=CARTESIAN_POINT ( 'NONE',  ( -20.71335220384823117, -27.86167394782616213, -16.50001200000000168 ) ) ;
#16816=ORIENTED_EDGE ( 'NONE', *, *, #29186, .F. ) ;
#16843=EDGE_LOOP ( 'NONE', ( #10525, #9554 ) ) ;
#16848=CARTESIAN_POINT ( 'NONE',  ( -39.52380524535560369, 7.028748154183623420, -6.500000000000000888 ) ) ;
#16855=AXIS2_PLACEMENT_3D ( 'NONE', #14240, #24070, #12228 ) ;
#16861=ORIENTED_EDGE ( 'NONE', *, *, #28246, .T. ) ;
#16871=SHAPE_REPRESENTATION ( 'Cartridge Outer Retaining Cylinder', ( #7396 ), #14351 ) ;
#16872=CARTESIAN_POINT ( 'NONE',  ( -26.41394434536854874, -32.09691347257047767, -6.500000000000000888 ) ) ;
#16878=CARTESIAN_POINT ( 'NONE',  ( -19.64114023396299302, -37.13592150529018454, -1.500000000000000000 ) ) ;
#16886=CARTESIAN_POINT ( 'NONE',  ( 39.00000000000000000, -5.563236990218592304, -1.500000000000000000 ) ) ;
#16888=VERTEX_POINT ( 'NONE', #3270 ) ;
#16929=ORIENTED_EDGE ( 'NONE', *, *, #24286, .T. ) ;
#16943=CARTESIAN_POINT ( 'NONE',  ( 2.075483152176834878, 44.03327996489939977, -16.50000000000000000 ) ) ;
#16988=FACE_OUTER_BOUND ( 'NONE', #10804, .T. ) ;
#16990=CARTESIAN_POINT ( 'NONE',  ( -32.82330813384395185, 22.94799032727105370, -1.500000000000000000 ) ) ;
#16996=ORIENTED_EDGE ( 'NONE', *, *, #6714, .F. ) ;
#17005=ORIENTED_EDGE ( 'NONE', *, *, #25211, .F. ) ;
#17008=UNCERTAINTY_MEASURE_WITH_UNIT (LENGTH_MEASURE( 1.000000000000000082E-05 ), #9640, 'distance_accuracy_value', 'NONE');
#17015=DIRECTION ( 'NONE',  ( -1.000000000000000000, 0.000000000000000000, 0.000000000000000000 ) ) ;
#17019=DIRECTION ( 'NONE',  ( 1.000000000000000000, 0.000000000000000000, 0.000000000000000000 ) ) ;
#17023=DIRECTION ( 'NONE',  ( 0.000000000000000000, 0.000000000000000000, -1.000000000000000000 ) ) ;
#17024=CARTESIAN_POINT ( 'NONE',  ( -25.19442432475474902, -35.44676296258422354, -19.50000000000000355 ) ) ;
#17028=EDGE_CURVE ( 'NONE', #20269, #2425, #5758, .T. ) ;
#17029=CARTESIAN_POINT ( 'NONE',  ( -32.51029856060266354, 26.37762524645828321, -16.50000000000000355 ) ) ;
#17034=CARTESIAN_POINT ( 'NONE',  ( -10.64374042650306862, 42.96126232887723972, -19.50000000000000355 ) ) ;
#17035=EDGE_CURVE ( 'NONE', #13676, #18657, #21605, .T. ) ;
#17048=ORIENTED_EDGE ( 'NONE', *, *, #2670, .F. ) ;
#17052=CARTESIAN_POINT ( 'NONE',  ( 12.33859880789482233, -8.132258305203423632, -1.500000000000000000 ) ) ;
#17053=CARTESIAN_POINT ( 'NONE',  ( -20.45518110071315832, 26.46109910111415786, -16.50001199999999812 ) ) ;
#17056=CARTESIAN_POINT ( 'NONE',  ( 11.83251621799620779, -42.16142857676437217, -16.50000000000000000 ) ) ;
#17093=CARTESIAN_POINT ( 'NONE',  ( 22.85913406299476591, 36.41590270059426615, -16.50000000000000000 ) ) ;
#17106=CARTESIAN_POINT ( 'NONE',  ( 0.000000000000000000, 0.000000000000000000, -16.50000000000000000 ) ) ;
#17127=VECTOR ( 'NONE', #14324, 1000.000000000000114 ) ;
#17141=EDGE_LOOP ( 'NONE', ( #21245, #9413 ) ) ;
#17151=CARTESIAN_POINT ( 'NONE',  ( 39.52380524535562500, 7.028748154183637631, -1.499999999999999556 ) ) ;
#17164=DIRECTION ( 'NONE',  ( -0.000000000000000000, -0.000000000000000000, -1.000000000000000000 ) ) ;
#17172=EDGE_CURVE ( 'NONE', #26111, #22154, #17708, .T. ) ;
#17177=CARTESIAN_POINT ( 'NONE',  ( 19.64114023396309960, -37.13592150529014191, -1.500000000000000000 ) ) ;
#17183=PLANE ( 'NONE',  #17319 ) ;
#17185=CARTESIAN_POINT ( 'NONE',  ( 4.336808689942017736E-16, 42.50000000000000000, -1.500000000000000000 ) ) ;
#17204=EDGE_CURVE ( 'NONE', #13692, #1863, #25353, .T. ) ;
#17244=ORIENTED_EDGE ( 'NONE', *, *, #22, .F. ) ;
#17250=CARTESIAN_POINT ( 'NONE',  ( 7.241839955191071709, 43.38385797512582087, -16.49999999999999645 ) ) ;
#17271=AXIS2_PLACEMENT_3D ( 'NONE', #797, #8299, #17340 ) ;
#17306=CARTESIAN_POINT ( 'NONE',  ( -25.64627119138473432, 23.40052582045089480, -6.500000000000000888 ) ) ;
#17319=AXIS2_PLACEMENT_3D ( 'NONE', #7833, #26704, #29194 ) ;
#17320=CARTESIAN_POINT ( 'NONE',  ( 20.71335220384823117, -27.86167394782616213, -16.50000600000000262 ) ) ;
#17328=LINE ( 'NONE', #9849, #3370 ) ;
#17340=DIRECTION ( 'NONE',  ( 1.000000000000000000, 0.000000000000000000, 0.000000000000000000 ) ) ;
#17343=B_SPLINE_SURFACE_WITH_KNOTS ( 'NONE', 1, 3, ( 
 ( #30021, #25172, #1170, #27532, #6305, #15819, #20036, #10843, #15350, #20350, #29879, #27215, #27384, #15978, #22522, #29708, #17697, #5851, #18169, #25337, #3979, #6005, #1639, #8801, #22983, #6153, #20646, #27840, #3519, #11150, #18327, #10677, #6468, #23135, #20183, #25499, #4124, #13651, #10999, #8520, #1781, #8192 ),
 ( #15508, #17867, #22671, #8352, #3666, #25024, #13180, #3817, #15659, #13340, #22837, #1488, #20498, #18481, #20940, #9562, #14078, #26244, #13792, #23741, #18626, #11920, #2393, #9258, #6760, #4575, #1932, #11457, #2075, #21411, #25647, #11749, #4884, #21243, #16578, #30319, #23586, #30464, #18937, #16278, #28137, #9108 ) ),
 .UNSPECIFIED., .F., .T., .F.,
 ( 2, 2 ),
 ( 4, 2, 2, 2, 2, 2, 2, 2, 2, 2, 2, 2, 2, 2, 2, 2, 2, 2, 2, 2, 4 ),
 ( 0.000000000000000000, 1.000000000000000000 ),
 ( 0.000000000000000000, 0.1963495408493620697, 0.3926990816987241395, 0.7853981633974482790, 1.178097245096172418, 1.570796326794896558, 1.963495408493620697, 2.356194490192344837, 2.748893571891068976, 2.945243112740430824, 3.141592653589793116, 3.337942194439155408, 3.534291735288517255, 3.926990816987241395, 4.319689898685965090, 4.712388980384689674, 5.105088062083414258, 5.497787143782137953, 5.890486225480861648, 6.086835766330223940, 6.283185307179586232 ),
 .UNSPECIFIED. ) ;
#17345=LINE ( 'NONE', #22790, #21720 ) ;
#17346=AXIS2_PLACEMENT_3D ( 'NONE', #522, #4901, #21579 ) ;
#17347=CARTESIAN_POINT ( 'NONE',  ( -5.374868878254082105, 44.10336124695542992, -19.50000000000000355 ) ) ;
#17348=DIRECTION ( 'NONE',  ( -0.000000000000000000, -0.000000000000000000, -1.000000000000000000 ) ) ;
#17353=CARTESIAN_POINT ( 'NONE',  ( 33.46566279634534169, -23.92259740141108537, -11.49999999999999822 ) ) ;
#17356=DIRECTION ( 'NONE',  ( -0.000000000000000000, 0.000000000000000000, 1.000000000000000000 ) ) ;
#17366=DIRECTION ( 'NONE',  ( -0.000000000000000000, -0.000000000000000000, 1.000000000000000000 ) ) ;
#17371=CARTESIAN_POINT ( 'NONE',  ( -20.64946329957944116, 25.40401715649331749, -16.50001200000000523 ) ) ;
#17373=ORIENTED_EDGE ( 'NONE', *, *, #4084, .T. ) ;
#17387=VERTEX_POINT ( 'NONE', #28581 ) ;
#17390=CARTESIAN_POINT ( 'NONE',  ( 39.83602371822922095, -11.57901747687539640, -19.50000000000000355 ) ) ;
#17456=DIRECTION ( 'NONE',  ( 0.5503133621338236470, -0.8349582046168341209, 0.000000000000000000 ) ) ;
#17505=CARTESIAN_POINT ( 'NONE',  ( -31.18700685316100163, -26.11823559932341610, -1.500000000000000000 ) ) ;
#17523=CARTESIAN_POINT ( 'NONE',  ( -23.91679456219655364, 22.99653376284463135, -16.50001200000000523 ) ) ;
#17537=CARTESIAN_POINT ( 'NONE',  ( 20.65888525914375862, -38.75220717792901581, -19.50000000000000355 ) ) ;
#17592=CARTESIAN_POINT ( 'NONE',  ( 40.57341518701483096, 0.5662347448574781561, -16.50000000000000000 ) ) ;
#17595=CARTESIAN_POINT ( 'NONE',  ( 39.87350638640253919, -4.706224724400470016, -11.49999999999999645 ) ) ;
#17600=CARTESIAN_POINT ( 'NONE',  ( 20.71335220384823117, -27.86167394782616213, -16.50001200000000168 ) ) ;
#17603=CARTESIAN_POINT ( 'NONE',  ( -33.13218612630368654, 7.028748154183637631, -1.942616967526160643 ) ) ;
#17604=ADVANCED_FACE ( 'NONE', ( #4673 ), #18714, .F. ) ;
#17610=ORIENTED_EDGE ( 'NONE', *, *, #24838, .F. ) ;
#17650=CARTESIAN_POINT ( 'NONE',  ( -31.18700685316050780, 26.11823559932051353, -1.500000000000000000 ) ) ;
#17670=CARTESIAN_POINT ( 'NONE',  ( 24.03057240117690441, -26.57182937991349903, -1.500000000000001332 ) ) ;
#17680=CYLINDRICAL_SURFACE ( 'NONE', #22086, 1.447898107987198646 ) ;
#17684=DIRECTION ( 'NONE',  ( 0.000000000000000000, -1.000000000000000000, 0.000000000000000000 ) ) ;
#17687=CARTESIAN_POINT ( 'NONE',  ( -23.00100564131931691, 35.20929533517665533, -8.166629612147223938 ) ) ;
#17697=CARTESIAN_POINT ( 'NONE',  ( 20.65888525914375862, -38.75220717792901581, -19.50000000000000355 ) ) ;
#17708=CIRCLE ( 'NONE', #15218, 27.70876437800068359 ) ;
#17709=LINE ( 'NONE', #27399, #2404 ) ;
#17712=CARTESIAN_POINT ( 'NONE',  ( -40.53232212831233028, -2.361325892396209714, -16.49999999999999645 ) ) ;
#17721=EDGE_LOOP ( 'NONE', ( #21009, #14189, #21632, #23378 ) ) ;
#17724=DIRECTION ( 'NONE',  ( -1.000000000000000000, 0.000000000000000000, 0.000000000000000000 ) ) ;
#17737=CARTESIAN_POINT ( 'NONE',  ( 40.35742903647388147, -4.708108710862773272, -16.50000000000000000 ) ) ;
#17747=B_SPLINE_CURVE_WITH_KNOTS ( 'NONE', 3,
 ( #828, #10351, #29684, #17053, #5671, #17371, #26585, #8021, #5209, #14710, #24217, #26895, #2867, #17523, #27044, #1300, #11126, #1908 ),
 .UNSPECIFIED., .F., .F.,
 ( 4, 2, 2, 2, 2, 2, 2, 2, 4 ),
 ( 0.000000000000000000, 0.1250000000000000000, 0.2500000000000000000, 0.3750000000000000000, 0.5000000000000000000, 0.6250000000000000000, 0.7500000000000000000, 0.8750000000000000000, 1.000000000000000000 ),
 .UNSPECIFIED. ) ;
#17764=CARTESIAN_POINT ( 'NONE',  ( -25.64627119138473788, 23.40052582045089480, -6.500000000000000888 ) ) ;
#17780=ADVANCED_FACE ( 'NONE', ( #6528 ), #3734, .F. ) ;
#17815=VECTOR ( 'NONE', #4589, 1000.000000000000114 ) ;
#17835=AXIS2_PLACEMENT_3D ( 'NONE', #25848, #4480, #25223 ) ;
#17848=AXIS2_PLACEMENT_3D ( 'NONE', #5297, #27136, #29158 ) ;
#17856=CARTESIAN_POINT ( 'NONE',  ( -20.65888525914099105, 38.75220717792564784, -19.50000000000000355 ) ) ;
#17862=CARTESIAN_POINT ( 'NONE',  ( 0.000000000000000000, 44.39187623478217404, -19.50000000000000355 ) ) ;
#17867=CARTESIAN_POINT ( 'NONE',  ( 2.552544031601107211, 42.49999999998228617, -1.500000000000000000 ) ) ;
#17872=VECTOR ( 'NONE', #8171, 1000.000000000000114 ) ;
#17889=DIRECTION ( 'NONE',  ( -0.5503133621338236470, -0.8349582046168341209, 0.000000000000000000 ) ) ;
#17900=CARTESIAN_POINT ( 'NONE',  ( 35.76344986165623396, 22.29344514668041199, -19.50000000000000355 ) ) ;
#17908=EDGE_CURVE ( 'NONE', #27870, #16473, #8283, .T. ) ;
#17944=EDGE_LOOP ( 'NONE', ( #19960, #9386, #19975, #25202, #13525, #12748, #6320, #9116 ) ) ;
#17946=CIRCLE ( 'NONE', #26919, 1.447898107987198646 ) ;
#17970=ORIENTED_EDGE ( 'NONE', *, *, #5564, .F. ) ;
#17986=CARTESIAN_POINT ( 'NONE',  ( 33.78553873773097393, 24.40792641592722134, -16.50000000000000000 ) ) ;
#17998=CARTESIAN_POINT ( 'NONE',  ( -20.64946329957944116, -25.40401715649331749, -16.50001200000000168 ) ) ;
#18001=FACE_OUTER_BOUND ( 'NONE', #29871, .T. ) ;
#18027=CARTESIAN_POINT ( 'NONE',  ( -32.24119420145671455, 26.76047160551536663, -16.50000600000000262 ) ) ;
#18040=CARTESIAN_POINT ( 'NONE',  ( 25.64627119138473432, 23.40052582045089480, -6.500000000000000888 ) ) ;
#18046=CARTESIAN_POINT ( 'NONE',  ( 2.687479362164894248, -44.39187623478217404, -19.50000000000000355 ) ) ;
#18051=DIRECTION ( 'NONE',  ( -0.000000000000000000, -0.000000000000000000, -1.000000000000000000 ) ) ;
#18061=VECTOR ( 'NONE', #10556, 1000.000000000000000 ) ;
#18074=PLANE ( 'NONE',  #13860 ) ;
#18117=DIRECTION ( 'NONE',  ( 1.000000000000000000, 0.000000000000000000, 0.000000000000000000 ) ) ;
#18145=CARTESIAN_POINT ( 'NONE',  ( -20.78475560873934569, -25.06838084537526612, -16.50001200000000523 ) ) ;
#18146=FACE_OUTER_BOUND ( 'NONE', #3721, .T. ) ;
#18159=CARTESIAN_POINT ( 'NONE',  ( 0.000000000000000000, 44.39187623478217404, -19.50000000000000355 ) ) ;
#18163=CARTESIAN_POINT ( 'NONE',  ( -20.65888525914099105, 38.75220717792564784, -19.50000000000000355 ) ) ;
#18169=CARTESIAN_POINT ( 'NONE',  ( 10.64374042650304020, -42.96126232887725394, -19.50000000000000355 ) ) ;
#18171=VECTOR ( 'NONE', #13425, 1000.000000000000114 ) ;
#18178=VERTEX_POINT ( 'NONE', #5205 ) ;
#18179=CARTESIAN_POINT ( 'NONE',  ( -31.61046531718546149, 26.43913157134711156, -9.833326303388901124 ) ) ;
#18180=EDGE_CURVE ( 'NONE', #13938, #24446, #14706, .T. ) ;
#18188=CARTESIAN_POINT ( 'NONE',  ( 26.41394434536444535, -32.09691347256665495, -6.500000000000000000 ) ) ;
#18198=CARTESIAN_POINT ( 'NONE',  ( 25.19442432474404470, 35.44676296256560022, -19.50000000000000355 ) ) ;
#18203=CARTESIAN_POINT ( 'NONE',  ( 23.22298176981586337, -35.92225146852586448, -14.83329738391580221 ) ) ;
#18220=DIRECTION ( 'NONE',  ( 0.9547931052914336858, 0.2972711322815274615, -0.000000000000000000 ) ) ;
#18230=ORIENTED_EDGE ( 'NONE', *, *, #22307, .F. ) ;
#18244=CARTESIAN_POINT ( 'NONE',  ( 0.000000000000000000, -7.028748154183644736, -16.50000000000000000 ) ) ;
#18257=ORIENTED_EDGE ( 'NONE', *, *, #24597, .T. ) ;
#18281=VERTEX_POINT ( 'NONE', #11123 ) ;
#18294=DIRECTION ( 'NONE',  ( 0.8349582046168341209, 0.5503133621338236470, 0.000000000000000000 ) ) ;
#18295=CARTESIAN_POINT ( 'NONE',  ( -22.94541271838176755, -35.03073867844241818, -6.500000000000000888 ) ) ;
#18319=CARTESIAN_POINT ( 'NONE',  ( 2.552544030762014415, -42.50000000000000000, -1.500000000000000000 ) ) ;
#18322=ADVANCED_FACE ( 'NONE', ( #4096 ), #15634, .F. ) ;
#18325=DIRECTION ( 'NONE',  ( 0.2972711322815266843, -0.9547931052914337968, -0.000000000000000000 ) ) ;
#18327=CARTESIAN_POINT ( 'NONE',  ( -40.89187623478217404, -5.790488632116337797, -19.50000000000000355 ) ) ;
#18369=EDGE_CURVE ( 'NONE', #6009, #3753, #20606, .T. ) ;
#18387=EDGE_CURVE ( 'NONE', #4045, #27870, #30589, .T. ) ;
#18394=CARTESIAN_POINT ( 'NONE',  ( -20.71335220384823117, 27.86167394782616213, -6.500000000000000888 ) ) ;
#18417=CARTESIAN_POINT ( 'NONE',  ( 25.64627119138473432, -23.40052582045089480, -6.500000000000000888 ) ) ;
#18431=CARTESIAN_POINT ( 'NONE',  ( 26.41394434536411140, 32.09691347256533334, -6.500000000000000888 ) ) ;
#18437=VERTEX_POINT ( 'NONE', #22308 ) ;
#18471=CARTESIAN_POINT ( 'NONE',  ( -5.105024945673440229, 42.22604126506271172, -1.500000000000000000 ) ) ;
#18472=CARTESIAN_POINT ( 'NONE',  ( 20.65888525914375862, -38.75220717792901581, -19.50000000000000355 ) ) ;
#18481=CARTESIAN_POINT ( 'NONE',  ( 34.07766914598172292, -21.40380666527112652, -1.500000000000000000 ) ) ;
#18486=CARTESIAN_POINT ( 'NONE',  ( -31.45274955338950207, 26.35877938683250576, -8.166661939820002658 ) ) ;
#18510=CARTESIAN_POINT ( 'NONE',  ( 39.00000000000000000, 5.563236990218597633, -1.500000000000000000 ) ) ;
#18523=ADVANCED_FACE ( 'NONE', ( #24648 ), #5479, .F. ) ;
#18551=VECTOR ( 'NONE', #20171, 1000.000000000000000 ) ;
#18557=VERTEX_POINT ( 'NONE', #25115 ) ;
#18562=ORIENTED_EDGE ( 'NONE', *, *, #22477, .T. ) ;
#18564=CARTESIAN_POINT ( 'NONE',  ( -22.58267429318970443, -26.57182937991348481, 26.54355021145563143 ) ) ;
#18567=AXIS2_PLACEMENT_3D ( 'NONE', #23838, #28381, #16515 ) ;
#18579=CARTESIAN_POINT ( 'NONE',  ( 0.000000000000000000, 0.000000000000000000, -16.50000000000000000 ) ) ;
#18580=CARTESIAN_POINT ( 'NONE',  ( -25.64627119138473432, -23.40052582045089480, -16.50000600000000262 ) ) ;
#18591=CARTESIAN_POINT ( 'NONE',  ( 39.52380524535562500, 7.028748154183637631, -6.500000000000000888 ) ) ;
#18601=CARTESIAN_POINT ( 'NONE',  ( -39.52380524536136619, -7.028748154183644736, -11.49999999999999645 ) ) ;
#18605=DIRECTION ( 'NONE',  ( -1.000000000000000000, 0.000000000000000000, 0.000000000000000000 ) ) ;
#18626=CARTESIAN_POINT ( 'NONE',  ( 2.552544030762014415, -42.50000000000000000, -1.500000000000000000 ) ) ;
#18635=VECTOR ( 'NONE', #2482, 1000.000000000000000 ) ;
#18652=ORIENTED_EDGE ( 'NONE', *, *, #11025, .T. ) ;
#18657=VERTEX_POINT ( 'NONE', #26936 ) ;
#18664=CARTESIAN_POINT ( 'NONE',  ( -23.27838112031802709, -36.10018649381529343, -16.50000600000000262 ) ) ;
#18677=B_SPLINE_CURVE_WITH_KNOTS ( 'NONE', 3,
 ( #5191, #347, #9870, #17353, #21875, #3165, #19387, #7841, #28905, #812 ),
 .UNSPECIFIED., .F., .F.,
 ( 4, 3, 3, 4 ),
 ( -0.005033671593837414984, 0.000000000000000000, 0.005033946531780188541, 0.01006789358107997023 ),
 .UNSPECIFIED. ) ;
#18692=DIRECTION ( 'NONE',  ( 0.2972711322815266288, -0.9547931052914337968, 0.000000000000000000 ) ) ;
#18714=PLANE ( 'NONE',  #11283 ) ;
#18720=CARTESIAN_POINT ( 'NONE',  ( 40.05104235265675783, 2.353288714459732311, -6.500000000000000888 ) ) ;
#18747=CARTESIAN_POINT ( 'NONE',  ( 32.51029956715037628, -26.37762564238233765, -16.50000000000000355 ) ) ;
#18757=CARTESIAN_POINT ( 'NONE',  ( 2.687479363073301819, 44.39187623479102740, -19.50000000000000355 ) ) ;
#18766=CARTESIAN_POINT ( 'NONE',  ( 4.336808689942017736E-16, 42.50000000000000000, -1.500000000000000000 ) ) ;
#18768=CARTESIAN_POINT ( 'NONE',  ( 20.65888525914559892, 38.75220717792412728, -19.50000000000000355 ) ) ;
#18775=CIRCLE ( 'NONE', #7819, 3.559164065751841743 ) ;
#18799=CARTESIAN_POINT ( 'NONE',  ( -39.52380524536133777, -7.028748154183623420, -6.500000000000000888 ) ) ;
#18801=DIRECTION ( 'NONE',  ( -0.000000000000000000, -0.000000000000000000, -1.000000000000000000 ) ) ;
#18804=CIRCLE ( 'NONE', #5350, 1.447898107987198646 ) ;
#18806=CARTESIAN_POINT ( 'NONE',  ( 29.55332031600788767, -27.89853503085224773, -1.500000000000000000 ) ) ;
#18811=CARTESIAN_POINT ( 'NONE',  ( 32.81350286003733885, 7.028748154183637631, -6.500000000000000888 ) ) ;
#18812=CARTESIAN_POINT ( 'NONE',  ( 4.336808689942017736E-16, 42.50000000000000000, -1.500000000000000000 ) ) ;
#18813=CARTESIAN_POINT ( 'NONE',  ( -22.94541271838176044, 35.03073867844246081, -6.500000000000000888 ) ) ;
#18815=AXIS2_PLACEMENT_3D ( 'NONE', #3795, #4242, #10816 ) ;
#18843=EDGE_LOOP ( 'NONE', ( #13170, #6002, #448, #29549 ) ) ;
#18869=VECTOR ( 'NONE', #2259, 1000.000000000000000 ) ;
#18885=CARTESIAN_POINT ( 'NONE',  ( -40.05104235265675783, 2.353288714454549790, -6.500000000000000888 ) ) ;
#18886=PRODUCT_DEFINITION_SHAPE ( 'NONE', 'NONE',  #2093 ) ;
#18892=CARTESIAN_POINT ( 'NONE',  ( 32.81350286003733885, -7.028748154183637631, -6.500000000000000888 ) ) ;
#18906=EDGE_CURVE ( 'NONE', #25162, #12583, #7087, .T. ) ;
#18918=CARTESIAN_POINT ( 'NONE',  ( 25.19442432473618254, -35.44676296258426618, -19.50000000000000355 ) ) ;
#18925=EDGE_CURVE ( 'NONE', #26229, #19866, #16743, .T. ) ;
#18931=EDGE_CURVE ( 'NONE', #16453, #8571, #28934, .T. ) ;
#18937=CARTESIAN_POINT ( 'NONE',  ( -10.11202017158466759, 41.14070756921185534, -1.500000000000000000 ) ) ;
#18953=CARTESIAN_POINT ( 'NONE',  ( 12.56641067637329812, 40.32935944495179115, -1.500000000000003997 ) ) ;
#18958=DIRECTION ( 'NONE',  ( -0.000000000000000000, 0.000000000000000000, -1.000000000000000000 ) ) ;
#18960=CARTESIAN_POINT ( 'NONE',  ( 26.80246859415415273, -7.028748154183637631, -1.499999999999999556 ) ) ;
#18969=CARTESIAN_POINT ( 'NONE',  ( 2.552544031601107211, 42.49999999998228617, -1.500000000000000000 ) ) ;
#18990=FACE_OUTER_BOUND ( 'NONE', #25309, .T. ) ;
#18993=DIRECTION ( 'NONE',  ( 0.000000000000000000, 0.000000000000000000, -1.000000000000000000 ) ) ;
#19027=DIRECTION ( 'NONE',  ( -0.000000000000000000, -0.000000000000000000, 1.000000000000000000 ) ) ;
#19030=CARTESIAN_POINT ( 'NONE',  ( -39.70095622561521509, -7.028748154183642072, -13.16666434783603989 ) ) ;
#19046=CARTESIAN_POINT ( 'NONE',  ( -18.48743143136275435, 39.23974440348072079, -16.50000000000000355 ) ) ;
#19057=CARTESIAN_POINT ( 'NONE',  ( 37.98493438989863336, -11.12428508576153341, -1.500000000000000000 ) ) ;
#19058=CARTESIAN_POINT ( 'NONE',  ( 39.52380524535562500, 7.028748154183637631, -11.49999999999999645 ) ) ;
#19075=EDGE_CURVE ( 'NONE', #20004, #26411, #8822, .T. ) ;
#19081=CARTESIAN_POINT ( 'NONE',  ( -24.03057240117691862, 26.57182937991348481, -1.500000000000001332 ) ) ;
#19092=CARTESIAN_POINT ( 'NONE',  ( 33.13218612630368654, 7.028748154183637631, -1.942616967526160643 ) ) ;
#19098=ORIENTED_EDGE ( 'NONE', *, *, #13501, .F. ) ;
#19109=CARTESIAN_POINT ( 'NONE',  ( 23.96732207938043402, -33.98584080152387088, -1.500000000000000000 ) ) ;
#19118=AXIS2_PLACEMENT_3D ( 'NONE', #24438, #2936, #3079 ) ;
#19129=CARTESIAN_POINT ( 'NONE',  ( 0.000000000000000000, 0.000000000000000000, -16.50000000000000000 ) ) ;
#19130=DIRECTION ( 'NONE',  ( -0.000000000000000000, -0.000000000000000000, -1.000000000000000000 ) ) ;
#19173=DIRECTION ( 'NONE',  ( 0.000000000000000000, 1.000000000000000000, 0.000000000000000000 ) ) ;
#19177=CARTESIAN_POINT ( 'NONE',  ( 40.05104235265675783, -2.353288714521559744, -6.500000000000000888 ) ) ;
#19204=CARTESIAN_POINT ( 'NONE',  ( 39.00000000000000000, 5.563236990218597633, -1.500000000000000000 ) ) ;
#19207=ORIENTED_EDGE ( 'NONE', *, *, #25631, .F. ) ;
#19208=FACE_OUTER_BOUND ( 'NONE', #12922, .T. ) ;
#19212=CARTESIAN_POINT ( 'NONE',  ( -32.74775157610409337, 27.21557300919391054, -19.50000000000000355 ) ) ;
#19213=ORIENTED_EDGE ( 'NONE', *, *, #17035, .F. ) ;
#19217=ORIENTED_EDGE ( 'NONE', *, *, #24212, .T. ) ;
#19226=ORIENTED_EDGE ( 'NONE', *, *, #7357, .T. ) ;
#19231=VECTOR ( 'NONE', #22332, 1000.000000000000000 ) ;
#19252=CARTESIAN_POINT ( 'NONE',  ( 12.56641067637628240, -40.32935944494942504, -1.500000000000000000 ) ) ;
#19258=CARTESIAN_POINT ( 'NONE',  ( 39.83602371821015709, 11.57901747687536265, -19.50000000000000355 ) ) ;
#19267=VECTOR ( 'NONE', #17366, 1000.000000000000000 ) ;
#19277=CARTESIAN_POINT ( 'NONE',  ( 25.47847050916410439, -26.57182937991349903, -1.500000000000001332 ) ) ;
#19278=CARTESIAN_POINT ( 'NONE',  ( 23.27838112219106392, 36.10018657900367600, -16.50000600000000262 ) ) ;
#19283=EDGE_CURVE ( 'NONE', #25580, #8889, #14400, .T. ) ;
#19296=DIRECTION ( 'NONE',  ( 0.000000000000000000, 0.000000000000000000, -1.000000000000000000 ) ) ;
#19300=ORIENTED_EDGE ( 'NONE', *, *, #92, .F. ) ;
#19353=CARTESIAN_POINT ( 'NONE',  ( 20.71335220384823117, 27.86167394782616213, -16.50001200000000168 ) ) ;
#19358=CARTESIAN_POINT ( 'NONE',  ( -33.25198513809938561, 23.59839681648617216, -8.166573414591429270 ) ) ;
#19360=DIRECTION ( 'NONE',  ( -0.000000000000000000, -0.000000000000000000, -1.000000000000000000 ) ) ;
#19367=CARTESIAN_POINT ( 'NONE',  ( 26.80246859415415273, -7.028748154183637631, -1.499999999999999556 ) ) ;
#19372=CARTESIAN_POINT ( 'NONE',  ( 13.22505861668195237, -42.10773672056998862, -19.50000000000000355 ) ) ;
#19373=VECTOR ( 'NONE', #20745, 1000.000000000000000 ) ;
#19379=CARTESIAN_POINT ( 'NONE',  ( -2.552544030762004645, -42.50000000000000000, -1.500000000000000000 ) ) ;
#19381=CARTESIAN_POINT ( 'NONE',  ( 0.000000000000000000, 0.000000000000000000, -1.500000000000000000 ) ) ;
#19387=CARTESIAN_POINT ( 'NONE',  ( 33.14492814497746309, -23.43596551657708105, -6.499906363187121450 ) ) ;
#19405=CARTESIAN_POINT ( 'NONE',  ( 22.54178090630008313, -36.64935163255146477, -16.50000000000000000 ) ) ;
#19434=DIRECTION ( 'NONE',  ( -0.000000000000000000, -0.000000000000000000, 1.000000000000000000 ) ) ;
#19436=DIRECTION ( 'NONE',  ( -0.000000000000000000, -0.000000000000000000, -1.000000000000000000 ) ) ;
#19437=CARTESIAN_POINT ( 'NONE',  ( -5.105024945675580739, -42.22604126506273303, -1.500000000000000000 ) ) ;
#19449=B_SPLINE_CURVE_WITH_KNOTS ( 'NONE', 3,
 ( #13756, #13911, #12032, #28108, #16242, #4235, #1902, #26064, #2355, #11885, #2047, #19046, #16704, #21380, #4542, #4850, #17, #9529, #6730, #21063, #25760, #28563, #11569, #14367, #30586, #9683, #16101, #25621, #4695, #6883, #9225 ),
 .UNSPECIFIED., .F., .F.,
 ( 4, 2, 1, 1, 2, 2, 1, 2, 2, 2, 2, 2, 1, 2, 2, 1, 2, 4 ),
 ( 0.4060398654371175087, 0.4089824111038223298, 0.4119249567705270954, 0.4178100481039366820, 0.4207525937706414476, 0.4222238666039939137, 0.4236951394373462687, 0.4295802307707560219, 0.4531205961043950348, 0.4648907787712145412, 0.4678333244379194178, 0.4707758701046242944, 0.4766609614380340476, 0.4825460527714438563, 0.4884311441048536095, 0.4943162354382634183, 0.4972587811049682949, 0.5002013267716731715 ),
 .UNSPECIFIED. ) ;
#19456=VERTEX_POINT ( 'NONE', #24415 ) ;
#19457=EDGE_CURVE ( 'NONE', #4264, #14731, #27395, .T. ) ;
#19459=EDGE_CURVE ( 'NONE', #14649, #5977, #14604, .T. ) ;
#19465=VECTOR ( 'NONE', #22915, 1000.000000000000000 ) ;
#19466=FACE_OUTER_BOUND ( 'NONE', #898, .T. ) ;
#19476=EDGE_CURVE ( 'NONE', #2130, #13676, #23655, .T. ) ;
#19478=EDGE_CURVE ( 'NONE', #6853, #20269, #21460, .T. ) ;
#19495=B_SPLINE_CURVE_WITH_KNOTS ( 'NONE', 3,
 ( #10968, #814, #12992, #20002, #17986 ),
 .UNSPECIFIED., .F., .F.,
 ( 4, 1, 4 ),
 ( 0.6430105143128194145, 0.6483083546374348582, 0.6536061949620504130 ),
 .UNSPECIFIED. ) ;
#19524=DIRECTION ( 'NONE',  ( -0.000000000000000000, -0.000000000000000000, 1.000000000000000000 ) ) ;
#19532=CARTESIAN_POINT ( 'NONE',  ( -34.07766914599911701, 21.40380666528009002, -1.500000000000000000 ) ) ;
#19564=DIRECTION ( 'NONE',  ( -0.000000000000000000, -0.000000000000000000, -1.000000000000000000 ) ) ;
#19575=PRODUCT_CONTEXT ( 'NONE', #9626, 'mechanical' ) ;
#19587=CARTESIAN_POINT ( 'NONE',  ( 11.79327001302698719, 42.17510997215990898, -16.50000000000000355 ) ) ;
#19592=DIRECTION ( 'NONE',  ( 0.000000000000000000, 0.000000000000000000, -1.000000000000000000 ) ) ;
#19600=VECTOR ( 'NONE', #29689, 999.9999999999998863 ) ;
#19607=VECTOR ( 'NONE', #471, 1000.000000000000114 ) ;
#19612=CARTESIAN_POINT ( 'NONE',  ( -25.64627119138473432, -23.40052582045089480, -16.50001200000000168 ) ) ;
#19614=CARTESIAN_POINT ( 'NONE',  ( 40.57663165180618847, 0.1223933743677056846, -16.50000000000000000 ) ) ;
#19638=CARTESIAN_POINT ( 'NONE',  ( -32.24119442679361214, -26.76047168400493703, -16.50000600000000262 ) ) ;
#19650=DIRECTION ( 'NONE',  ( -0.000000000000000000, -0.000000000000000000, -1.000000000000000000 ) ) ;
#19652=ORIENTED_EDGE ( 'NONE', *, *, #21005, .F. ) ;
#19660=DIRECTION ( 'NONE',  ( 0.000000000000000000, 0.000000000000000000, -1.000000000000000000 ) ) ;
#19661=EDGE_CURVE ( 'NONE', #24153, #14363, #15195, .T. ) ;
#19675=CARTESIAN_POINT ( 'NONE',  ( -40.89187623478217404, 5.790488632116478129, -19.50000000000000355 ) ) ;
#19679=EDGE_CURVE ( 'NONE', #11174, #11716, #6477, .T. ) ;
#19681=ORIENTED_EDGE ( 'NONE', *, *, #28902, .F. ) ;
#19692=DIRECTION ( 'NONE',  ( 0.000000000000000000, 0.000000000000000000, -1.000000000000000000 ) ) ;
#19711=DIRECTION ( 'NONE',  ( 0.5503133621338236470, 0.8349582046168341209, 0.000000000000000000 ) ) ;
#19718=FACE_OUTER_BOUND ( 'NONE', #24906, .T. ) ;
#19726=EDGE_LOOP ( 'NONE', ( #21503, #20891, #8623, #4269 ) ) ;
#19728=DIRECTION ( 'NONE',  ( -1.000000000000000000, 0.000000000000000000, 0.000000000000000000 ) ) ;
#19732=FACE_BOUND ( 'NONE', #12973, .T. ) ;
#19735=VECTOR ( 'NONE', #20478, 1000.000000000000000 ) ;
#19776=CIRCLE ( 'NONE', #23268, 27.70876437800068359 ) ;
#19784=B_SPLINE_CURVE_WITH_KNOTS ( 'NONE', 3,
 ( #10697, #8210, #24574, #17712, #25045, #22239, #5869, #5709, #20203, #10399, #15369, #13053, #22544 ),
 .UNSPECIFIED., .F., .F.,
 ( 4, 2, 2, 2, 1, 2, 4 ),
 ( 0.2233868814791938606, 0.2366521944267142574, 0.2499175073742346820, 0.2532338356111147881, 0.2565501638479948943, 0.2631828203217550510, 0.2764481332692754756 ),
 .UNSPECIFIED. ) ;
#19822=CARTESIAN_POINT ( 'NONE',  ( 31.45274955328486399, 26.35877938677919374, -8.166661938643251517 ) ) ;
#19840=CARTESIAN_POINT ( 'NONE',  ( -2.687479363073305372, 44.39187623477332068, -19.50000000000000355 ) ) ;
#19853=EDGE_CURVE ( 'NONE', #8048, #8571, #2405, .T. ) ;
#19866=VERTEX_POINT ( 'NONE', #14709 ) ;
#19868=LINE ( 'NONE', #1302, #17872 ) ;
#19880=CARTESIAN_POINT ( 'NONE',  ( 19.64114023396890829, 37.13592150528549496, -1.500000000000000000 ) ) ;
#19903=CARTESIAN_POINT ( 'NONE',  ( 24.03057240117691862, 26.57182937991349903, -6.500000000000000888 ) ) ;
#19934=FACE_OUTER_BOUND ( 'NONE', #6452, .T. ) ;
#19960=ORIENTED_EDGE ( 'NONE', *, *, #19457, .F. ) ;
#19975=ORIENTED_EDGE ( 'NONE', *, *, #18931, .T. ) ;
#20002=CARTESIAN_POINT ( 'NONE',  ( 33.53984941789958896, 24.80927308773734197, -16.50000000000000355 ) ) ;
#20004=VERTEX_POINT ( 'NONE', #13006 ) ;
#20016=DIRECTION ( 'NONE',  ( -0.000000000000000000, -0.000000000000000000, -1.000000000000000000 ) ) ;
#20031=CARTESIAN_POINT ( 'NONE',  ( 39.00000000000000000, 5.563236990218597633, -1.500000000000000000 ) ) ;
#20036=CARTESIAN_POINT ( 'NONE',  ( 25.19442432474404470, 35.44676296256560022, -19.50000000000000355 ) ) ;
#20043=ORIENTED_EDGE ( 'NONE', *, *, #16434, .T. ) ;
#20044=PLANE ( 'NONE',  #4905 ) ;
#20070=CARTESIAN_POINT ( 'NONE',  ( 10.64374042650142904, 42.96126232887663576, -19.50000000000000355 ) ) ;
#20072=EDGE_CURVE ( 'NONE', #14363, #16328, #27778, .T. ) ;
#20074=DIRECTION ( 'NONE',  ( -1.000000000000000000, 0.000000000000000000, 0.000000000000000000 ) ) ;
#20083=CARTESIAN_POINT ( 'NONE',  ( 40.05520497557499482, 7.028746409576331011, -16.50000000000000000 ) ) ;
#20092=DIRECTION ( 'NONE',  ( -0.2972711322815274060, 0.9547931052914335748, 0.000000000000000000 ) ) ;
#20109=VERTEX_POINT ( 'NONE', #24176 ) ;
#20117=ORIENTED_EDGE ( 'NONE', *, *, #19459, .T. ) ;
#20123=AXIS2_PLACEMENT_3D ( 'NONE', #46, #14221, #27835 ) ;
#20126=CIRCLE ( 'NONE', #8111, 1.447898107987198646 ) ;
#20133=CARTESIAN_POINT ( 'NONE',  ( -39.87350638641265732, -4.706224724266450998, -6.500000000000000888 ) ) ;
#20152=CARTESIAN_POINT ( 'NONE',  ( 24.03057240117691862, 26.57182937991349903, 26.54355021145563143 ) ) ;
#20171=DIRECTION ( 'NONE',  ( 0.000000000000000000, -1.000000000000000000, 0.000000000000000000 ) ) ;
#20173=CARTESIAN_POINT ( 'NONE',  ( -32.74775157610409337, 27.21557300919391054, -19.50000000000000355 ) ) ;
#20183=CARTESIAN_POINT ( 'NONE',  ( -32.74775157610409337, 27.21557300919391054, -19.50000000000000355 ) ) ;
#20192=DIRECTION ( 'NONE',  ( 0.8910248307962438385, 0.4539545692076743522, 0.000000000000000000 ) ) ;
#20203=CARTESIAN_POINT ( 'NONE',  ( -40.53864323030092720, 2.051443709366309154, -16.50000000000000355 ) ) ;
#20240=EDGE_CURVE ( 'NONE', #5019, #5438, #14751, .T. ) ;
#20244=FACE_OUTER_BOUND ( 'NONE', #16650, .T. ) ;
#20269=VERTEX_POINT ( 'NONE', #12814 ) ;
#20306=CIRCLE ( 'NONE', #4350, 3.559164065751841743 ) ;
#20311=EDGE_CURVE ( 'NONE', #4151, #30377, #4311, .T. ) ;
#20319=VERTEX_POINT ( 'NONE', #11831 ) ;
#20338=CARTESIAN_POINT ( 'NONE',  ( -13.22505861668184046, -42.10773672057003125, -19.50000000000000355 ) ) ;
#20339=CARTESIAN_POINT ( 'NONE',  ( -23.22298176981137274, 35.92225146851140494, -14.83329738373930340 ) ) ;
#20344=CARTESIAN_POINT ( 'NONE',  ( -39.00000000000000000, -5.563236990218529243, -1.500000000000000000 ) ) ;
#20350=CARTESIAN_POINT ( 'NONE',  ( 39.83602371821015709, 11.57901747687536265, -19.50000000000000355 ) ) ;
#20378=VECTOR ( 'NONE', #18325, 1000.000000000000114 ) ;
#20385=VECTOR ( 'NONE', #12644, 1000.000000000000000 ) ;
#20413=ADVANCED_FACE ( 'NONE', ( #19934 ), #730, .T. ) ;
#20457=EDGE_CURVE ( 'NONE', #23101, #7851, #25533, .T. ) ;
#20461=DIRECTION ( 'NONE',  ( 0.000000000000000000, -0.000000000000000000, -1.000000000000000000 ) ) ;
#20478=DIRECTION ( 'NONE',  ( -0.000000000000000000, -0.000000000000000000, -1.000000000000000000 ) ) ;
#20493=CARTESIAN_POINT ( 'NONE',  ( -10.64374042650306862, 42.96126232887723972, -19.50000000000000355 ) ) ;
#20498=CARTESIAN_POINT ( 'NONE',  ( 37.98493438989863336, -11.12428508576153341, -1.500000000000000000 ) ) ;
#20509=FACE_BOUND ( 'NONE', #14852, .T. ) ;
#20526=CARTESIAN_POINT ( 'NONE',  ( 2.687479363073301819, 44.39187623479102740, -19.50000000000000355 ) ) ;
#20528=ORIENTED_EDGE ( 'NONE', *, *, #8916, .T. ) ;
#20531=CYLINDRICAL_SURFACE ( 'NONE', #27360, 7.500000000000000000 ) ;
#20537=CARTESIAN_POINT ( 'NONE',  ( 5.204170427930421283E-15, -44.07656352898514740, -16.50000000000000000 ) ) ;
#20543=AXIS2_PLACEMENT_3D ( 'NONE', #23770, #1961, #13819 ) ;
#20587=CARTESIAN_POINT ( 'NONE',  ( 20.71335220384823117, -27.86167394782616213, -6.500000000000000888 ) ) ;
#20598=CARTESIAN_POINT ( 'NONE',  ( 20.46975788395958418, -26.57181885929544407, -16.50000600000000262 ) ) ;
#20605=VECTOR ( 'NONE', #10524, 1000.000000000000114 ) ;
#20606=B_SPLINE_CURVE_WITH_KNOTS ( 'NONE', 3,
 ( #2050, #23879, #14052, #11572, #16707, #18601 ),
 .UNSPECIFIED., .F., .F.,
 ( 4, 2, 4 ),
 ( 1.408367944312347353, 1.570796326794896558, 1.733224709277445763 ),
 .UNSPECIFIED. ) ;
#20641=CARTESIAN_POINT ( 'NONE',  ( 13.22505861668195237, -42.10773672056998862, -19.50000000000000355 ) ) ;
#20646=CARTESIAN_POINT ( 'NONE',  ( -25.19442432475474902, -35.44676296258422354, -19.50000000000000355 ) ) ;
#20647=CARTESIAN_POINT ( 'NONE',  ( 26.80246859415415273, 7.028748154183637631, -1.499999999999999556 ) ) ;
#20670=LINE ( 'NONE', #6491, #7099 ) ;
#20674=CARTESIAN_POINT ( 'NONE',  ( -2.687479362164884034, -44.39187623478217404, -19.50000000000000355 ) ) ;
#20700=DIRECTION ( 'NONE',  ( 0.000000000000000000, -0.000000000000000000, -1.000000000000000000 ) ) ;
#20705=ORIENTED_EDGE ( 'NONE', *, *, #13192, .T. ) ;
#20706=CARTESIAN_POINT ( 'NONE',  ( 23.27838112219106392, 36.10018657900367600, -16.50000600000000262 ) ) ;
#20745=DIRECTION ( 'NONE',  ( -0.000000000000000000, -0.000000000000000000, -1.000000000000000000 ) ) ;
#20760=VECTOR ( 'NONE', #14382, 1000.000000000000000 ) ;
#20783=CARTESIAN_POINT ( 'NONE',  ( 32.74775157612609178, -27.21557300919356948, -19.50000000000000355 ) ) ;
#20787=CYLINDRICAL_SURFACE ( 'NONE', #20123, 1.447898107987198646 ) ;
#20803=CARTESIAN_POINT ( 'NONE',  ( -31.92585768991387951, 26.59981599196575175, -13.16665969541612036 ) ) ;
#20804=CIRCLE ( 'NONE', #13350, 7.500000000000000000 ) ;
#20829=CARTESIAN_POINT ( 'NONE',  ( 33.25198511596216377, 23.59839678289867493, -8.166573069426201315 ) ) ;
#20830=CARTESIAN_POINT ( 'NONE',  ( 10.11202017158463917, -41.14070756921186955, -1.500000000000000000 ) ) ;
#20831=ADVANCED_FACE ( 'NONE', ( #24334 ), #9837, .T. ) ;
#20851=ORIENTED_EDGE ( 'NONE', *, *, #18369, .F. ) ;
#20867=EDGE_LOOP ( 'NONE', ( #28536, #11264, #24388, #27386 ) ) ;
#20872=CIRCLE ( 'NONE', #9925, 27.70876437800068359 ) ;
#20891=ORIENTED_EDGE ( 'NONE', *, *, #24013, .T. ) ;
#20906=CARTESIAN_POINT ( 'NONE',  ( -26.80246859415415273, -7.028748154183637631, -6.500000000000000888 ) ) ;
#20917=ORIENTED_EDGE ( 'NONE', *, *, #26014, .F. ) ;
#20920=CARTESIAN_POINT ( 'NONE',  ( -20.58367780861512841, -27.52817754551177742, -16.50001200000000168 ) ) ;
#20926=CARTESIAN_POINT ( 'NONE',  ( 10.64374042650142904, 42.96126232887663576, -19.50000000000000355 ) ) ;
#20931=CARTESIAN_POINT ( 'NONE',  ( -5.105024945675580739, -42.22604126506273303, -1.500000000000000000 ) ) ;
#20940=CARTESIAN_POINT ( 'NONE',  ( 31.18700685317022803, -26.11823559933272421, -1.500000000000000000 ) ) ;
#20944=ORIENTED_EDGE ( 'NONE', *, *, #29217, .T. ) ;
#20983=VECTOR ( 'NONE', #11477, 1000.000000000000114 ) ;
#20991=CARTESIAN_POINT ( 'NONE',  ( -39.87350638641186862, -4.706224724276806270, -6.500000000000000888 ) ) ;
#20994=EDGE_CURVE ( 'NONE', #28062, #18437, #14808, .T. ) ;
#20996=CARTESIAN_POINT ( 'NONE',  ( 12.08030320849306527, -42.07844615544671996, -16.50000000000000355 ) ) ;
#21005=EDGE_CURVE ( 'NONE', #2231, #23836, #4657, .T. ) ;
#21009=ORIENTED_EDGE ( 'NONE', *, *, #27487, .F. ) ;
#21014=DIRECTION ( 'NONE',  ( 1.000000000000000000, 0.000000000000000000, 0.000000000000000000 ) ) ;
#21058=ORIENTED_EDGE ( 'NONE', *, *, #30517, .F. ) ;
#21063=CARTESIAN_POINT ( 'NONE',  ( -8.049211243008397076, 43.20179514148429689, -16.50000000000000000 ) ) ;
#21069=CARTESIAN_POINT ( 'NONE',  ( -22.21046885174908070, -23.49239644259612447, -16.50001200000000523 ) ) ;
#21082=CARTESIAN_POINT ( 'NONE',  ( -34.07766914599908148, -21.40380666528021081, -1.500000000000000000 ) ) ;
#21107=CARTESIAN_POINT ( 'NONE',  ( 33.78553873773097393, 24.40792641592722134, -16.50000000000000000 ) ) ;
#21113=CARTESIAN_POINT ( 'NONE',  ( -35.78163722268750746, 27.43648963448195133, -1.500000000000000000 ) ) ;
#21118=VERTEX_POINT ( 'NONE', #23829 ) ;
#21122=CARTESIAN_POINT ( 'NONE',  ( 19.64114023396890829, 37.13592150528549496, -1.500000000000000000 ) ) ;
#21127=EDGE_CURVE ( 'NONE', #18437, #8048, #4968, .T. ) ;
#21131=CARTESIAN_POINT ( 'NONE',  ( -7.256763913191261572, -43.38079396975989965, -16.50000000000000000 ) ) ;
#21143=CARTESIAN_POINT ( 'NONE',  ( 1.048387430112781127, -44.07656352898515451, -16.50000000000000355 ) ) ;
#21152=CARTESIAN_POINT ( 'NONE',  ( -39.52380524535562500, 7.028748154183637631, -11.49999999999999645 ) ) ;
#21183=CARTESIAN_POINT ( 'NONE',  ( 26.80246859415415273, -7.028748154183637631, -1.499999999999999556 ) ) ;
#21190=FACE_OUTER_BOUND ( 'NONE', #29714, .T. ) ;
#21201=DIRECTION ( 'NONE',  ( -1.000000000000000000, 0.000000000000000000, 0.000000000000000000 ) ) ;
#21224=CARTESIAN_POINT ( 'NONE',  ( 19.64114023396890829, 37.13592150528549496, -1.500000000000000000 ) ) ;
#21226=ORIENTED_EDGE ( 'NONE', *, *, #27289, .F. ) ;
#21240=EDGE_LOOP ( 'NONE', ( #6644, #14899, #23538, #10184 ) ) ;
#21243=CARTESIAN_POINT ( 'NONE',  ( -34.07766914599911701, 21.40380666528009002, -1.500000000000000000 ) ) ;
#21245=ORIENTED_EDGE ( 'NONE', *, *, #26838, .T. ) ;
#21259=CARTESIAN_POINT ( 'NONE',  ( 23.96732207937828463, 33.98584080152456011, -1.500000000000003997 ) ) ;
#21267=VECTOR ( 'NONE', #19027, 1000.000000000000000 ) ;
#21270=CARTESIAN_POINT ( 'NONE',  ( 25.64627119138473432, 23.40052582045089480, -16.50001200000000168 ) ) ;
#21271=CARTESIAN_POINT ( 'NONE',  ( 20.71335220384823117, -27.86167394782616213, -6.500000000000000888 ) ) ;
#21276=AXIS2_PLACEMENT_3D ( 'NONE', #19353, #9998, #21676 ) ;
#21283=CARTESIAN_POINT ( 'NONE',  ( -5.105024945673440229, 42.22604126506271172, -1.500000000000000000 ) ) ;
#21307=CARTESIAN_POINT ( 'NONE',  ( -39.52380524535562500, 7.028748154183637631, -11.49999999999999645 ) ) ;
#21316=VECTOR ( 'NONE', #13808, 999.9999999999998863 ) ;
#21346=CARTESIAN_POINT ( 'NONE',  ( -32.81350286003733885, 0.000000000000000000, -6.500000000000000888 ) ) ;
#21360=CARTESIAN_POINT ( 'NONE',  ( -2.552544031601109875, 42.50000000001772804, -1.500000000000009992 ) ) ;
#21363=PRODUCT ( 'Cartridge Outer Retaining Cylinder', 'Cartridge Outer Retaining Cylinder', '', ( #19575 ) ) ;
#21370=ORIENTED_EDGE ( 'NONE', *, *, #18180, .T. ) ;
#21380=CARTESIAN_POINT ( 'NONE',  ( -14.26810496549984997, 41.32347559458636255, -16.50000000000000355 ) ) ;
#21390=EDGE_CURVE ( 'NONE', #8048, #23566, #1408, .T. ) ;
#21392=CARTESIAN_POINT ( 'NONE',  ( 37.98493438987956949, 11.12428508576150143, -1.500000000000000000 ) ) ;
#21411=CARTESIAN_POINT ( 'NONE',  ( -37.98493438988125348, -11.12428508575252728, -1.500000000000000000 ) ) ;
#21436=CARTESIAN_POINT ( 'NONE',  ( 24.03057240117690441, -26.57182937991349903, -6.499999999999999112 ) ) ;
#21442=CARTESIAN_POINT ( 'NONE',  ( 33.57242512142757818, 24.08458161877725701, -13.16663720014176775 ) ) ;
#21443=CARTESIAN_POINT ( 'NONE',  ( -12.56641067637752229, 40.32935944495016400, -1.500000000000000000 ) ) ;
#21452=CARTESIAN_POINT ( 'NONE',  ( -33.46566279634666330, -23.92259740141309976, -11.50000000000000000 ) ) ;
#21453=DIRECTION ( 'NONE',  ( 0.8910248307962433945, -0.4539545692076750738, 0.000000000000000000 ) ) ;
#21458=CARTESIAN_POINT ( 'NONE',  ( -26.80246859415414917, -7.028748154183644736, -16.50000000000000000 ) ) ;
#21460=LINE ( 'NONE', #102, #11359 ) ;
#21464=FACE_BOUND ( 'NONE', #28078, .T. ) ;
#21485=DIRECTION ( 'NONE',  ( 0.9975640502598243087, 0.000000000000000000, 0.06975647374412531632 ) ) ;
#21491=DIRECTION ( 'NONE',  ( -0.000000000000000000, -0.000000000000000000, -1.000000000000000000 ) ) ;
#21503=ORIENTED_EDGE ( 'NONE', *, *, #20457, .T. ) ;
#21508=CARTESIAN_POINT ( 'NONE',  ( -39.87350638640939593, 4.706224724266459880, -6.500000000000000888 ) ) ;
#21518=DIRECTION ( 'NONE',  ( -1.000000000000000000, 0.000000000000000000, 0.000000000000000000 ) ) ;
#21523=CARTESIAN_POINT ( 'NONE',  ( -33.35889463998628912, 23.76060433659045046, -9.833271769321862976 ) ) ;
#21526=ORIENTED_EDGE ( 'NONE', *, *, #18387, .T. ) ;
#21534=CARTESIAN_POINT ( 'NONE',  ( 33.03678844028523542, -25.60268484000898681, -16.50000000000000000 ) ) ;
#21540=CARTESIAN_POINT ( 'NONE',  ( 10.11202017158463917, -41.14070756921186955, -1.500000000000000000 ) ) ;
#21548=CARTESIAN_POINT ( 'NONE',  ( 19.64114023396309960, -37.13592150529014191, -1.500000000000000000 ) ) ;
#21559=DIRECTION ( 'NONE',  ( -0.000000000000000000, -0.000000000000000000, -1.000000000000000000 ) ) ;
#21564=ADVANCED_FACE ( 'NONE', ( #9467 ), #21767, .T. ) ;
#21579=DIRECTION ( 'NONE',  ( 1.000000000000000000, 0.000000000000000000, 0.000000000000000000 ) ) ;
#21592=CARTESIAN_POINT ( 'NONE',  ( 2.552544030762014415, -42.50000000000000000, -1.500000000000000000 ) ) ;
#21605=B_SPLINE_CURVE_WITH_KNOTS ( 'NONE', 3,
 ( #11638, #4762, #30502, #9147, #30649, #2440, #21452, #546, #10068, #401 ),
 .UNSPECIFIED., .F., .F.,
 ( 4, 3, 3, 4 ),
 ( 2.017013542443209820E-16, 0.005033946524314806929, 0.01006789357361620452, 0.01510156516372195695 ),
 .UNSPECIFIED. ) ;
#21610=CARTESIAN_POINT ( 'NONE',  ( -19.82881186446047295, -38.45831515674161949, -16.50000000000000355 ) ) ;
#21628=FACE_OUTER_BOUND ( 'NONE', #3404, .T. ) ;
#21632=ORIENTED_EDGE ( 'NONE', *, *, #30561, .T. ) ;
#21645=CARTESIAN_POINT ( 'NONE',  ( -25.23756106473024019, 11.43858098102958287, -1.500000000000000000 ) ) ;
#21646=EDGE_LOOP ( 'NONE', ( #14291, #12749, #29258, #30045, #24505, #27170, #2227 ) ) ;
#21662=EDGE_LOOP ( 'NONE', ( #26917, #3125, #20117, #7188 ) ) ;
#21664=PLANE ( 'NONE',  #25266 ) ;
#21676=DIRECTION ( 'NONE',  ( 0.2972711322815261292, 0.9547931052914340189, 0.000000000000000000 ) ) ;
#21687=DIRECTION ( 'NONE',  ( -1.000000000000000000, 0.000000000000000000, 0.000000000000000000 ) ) ;
#21692=CARTESIAN_POINT ( 'NONE',  ( -39.00000000000000000, -5.563236990218529243, -1.500000000000000000 ) ) ;
#21700=CARTESIAN_POINT ( 'NONE',  ( 10.11202017158463917, -41.14070756921186955, -1.500000000000000000 ) ) ;
#21720=VECTOR ( 'NONE', #25132, 999.9999999999998863 ) ;
#21728=CARTESIAN_POINT ( 'NONE',  ( 5.204170427930421283E-15, -44.07656352898514740, -16.50000000000000000 ) ) ;
#21746=DIRECTION ( 'NONE',  ( -1.000000000000000000, 0.000000000000000000, 0.000000000000000000 ) ) ;
#21767=CYLINDRICAL_SURFACE ( 'NONE', #6857, 27.70876437800068359 ) ;
#21794=ADVANCED_FACE ( 'NONE', ( #19732, #10850 ), #20044, .T. ) ;
#21797=FACE_OUTER_BOUND ( 'NONE', #24879, .T. ) ;
#21809=CARTESIAN_POINT ( 'NONE',  ( 31.76816150359531576, -26.51947378167971792, -11.49999299985452694 ) ) ;
#21814=AXIS2_PLACEMENT_3D ( 'NONE', #2995, #19660, #29184 ) ;
#21830=LINE ( 'NONE', #17306, #19607 ) ;
#21833=ORIENTED_EDGE ( 'NONE', *, *, #21127, .F. ) ;
#21856=CARTESIAN_POINT ( 'NONE',  ( 26.80246859415415273, 7.028748154183637631, -16.50000000000000000 ) ) ;
#21858=ORIENTED_EDGE ( 'NONE', *, *, #24280, .F. ) ;
#21861=CARTESIAN_POINT ( 'NONE',  ( -40.89187623478217404, -5.790488632116337797, -19.50000000000000355 ) ) ;
#21864=VERTEX_POINT ( 'NONE', #6313 ) ;
#21869=CARTESIAN_POINT ( 'NONE',  ( -19.64114023396299302, -37.13592150529018454, -1.500000000000000000 ) ) ;
#21875=CARTESIAN_POINT ( 'NONE',  ( 33.35889463998532278, -23.76060433658897963, -9.833271769321870082 ) ) ;
#21880=ORIENTED_EDGE ( 'NONE', *, *, #649, .T. ) ;
#21882=CARTESIAN_POINT ( 'NONE',  ( 22.94541271837968566, 35.03073867843525591, -6.499999999999999112 ) ) ;
#21890=VECTOR ( 'NONE', #8966, 1000.000000000000000 ) ;
#21902=LINE ( 'NONE', #21271, #5313 ) ;
#21924=CARTESIAN_POINT ( 'NONE',  ( -12.56641067637617759, -40.32935944494947478, -1.500000000000000000 ) ) ;
#21935=CARTESIAN_POINT ( 'NONE',  ( 24.03057240117691862, -26.57182937991349903, -6.500000000000000888 ) ) ;
#21940=EDGE_CURVE ( 'NONE', #1863, #18281, #16636, .T. ) ;
#21993=EDGE_CURVE ( 'NONE', #26065, #6853, #30794, .T. ) ;
#22017=CARTESIAN_POINT ( 'NONE',  ( -23.96732207938974213, -33.98584080153308662, -1.500000000000000000 ) ) ;
#22031=ORIENTED_EDGE ( 'NONE', *, *, #5780, .T. ) ;
#22066=CARTESIAN_POINT ( 'NONE',  ( 0.000000000000000000, 0.000000000000000000, -16.50000000000000000 ) ) ;
#22083=DIRECTION ( 'NONE',  ( 0.000000000000000000, 0.000000000000000000, -1.000000000000000000 ) ) ;
#22086=AXIS2_PLACEMENT_3D ( 'NONE', #27048, #20016, #27198 ) ;
#22101=EDGE_CURVE ( 'NONE', #14088, #6009, #5978, .T. ) ;
#22104=CARTESIAN_POINT ( 'NONE',  ( 40.53905774364188375, 2.041855955180682081, -16.50000000000000355 ) ) ;
#22129=CARTESIAN_POINT ( 'NONE',  ( 25.64627119138473432, -23.40052582045089480, -16.50000000000000000 ) ) ;
#22138=LINE ( 'NONE', #17151, #20385 ) ;
#22148=EDGE_CURVE ( 'NONE', #13692, #28753, #3662, .T. ) ;
#22150=B_SPLINE_CURVE_WITH_KNOTS ( 'NONE', 3,
 ( #24479, #762, #15260, #15115, #10286, #7645, #19638 ),
 .UNSPECIFIED., .F., .F.,
 ( 4, 3, 4 ),
 ( 0.000000000000000000, 0.005028111721406030438, 0.01005622344633218777 ),
 .UNSPECIFIED. ) ;
#22154=VERTEX_POINT ( 'NONE', #13796 ) ;
#22172=CARTESIAN_POINT ( 'NONE',  ( 32.24119409414369386, 26.76047229433004659, -16.50000600000000262 ) ) ;
#22174=CARTESIAN_POINT ( 'NONE',  ( 5.105024945674004222, 42.22604126506330857, -1.500000000000000000 ) ) ;
#22201=EDGE_CURVE ( 'NONE', #17387, #4972, #484, .T. ) ;
#22208=CARTESIAN_POINT ( 'NONE',  ( 10.11202017158399968, 41.14070756921128691, -1.500000000000000000 ) ) ;
#22239=CARTESIAN_POINT ( 'NONE',  ( -40.57664911653668582, 0.2791883433268081416, -16.50000000000000000 ) ) ;
#22288=ORIENTED_EDGE ( 'NONE', *, *, #15674, .F. ) ;
#22304=CARTESIAN_POINT ( 'NONE',  ( -25.64627119138473432, -23.40052582045089480, -6.500000000000000888 ) ) ;
#22307=EDGE_CURVE ( 'NONE', #6254, #14731, #1260, .T. ) ;
#22308=CARTESIAN_POINT ( 'NONE',  ( 25.23756106473024019, 11.43858098102958287, -16.50000000000000000 ) ) ;
#22332=DIRECTION ( 'NONE',  ( -0.000000000000000000, -0.000000000000000000, -1.000000000000000000 ) ) ;
#22339=ORIENTED_EDGE ( 'NONE', *, *, #1199, .T. ) ;
#22371=CARTESIAN_POINT ( 'NONE',  ( -39.83602371821034183, 11.57901747687032490, -19.50000000000000355 ) ) ;
#22375=ORIENTED_EDGE ( 'NONE', *, *, #28026, .T. ) ;
#22377=CARTESIAN_POINT ( 'NONE',  ( -35.76344986165608475, 22.29344514668535027, -19.50000000000000355 ) ) ;
#22423=ORIENTED_EDGE ( 'NONE', *, *, #27078, .T. ) ;
#22437=DIRECTION ( 'NONE',  ( -0.4539545692076750738, -0.8910248307962433945, 0.000000000000000000 ) ) ;
#22438=ORIENTED_EDGE ( 'NONE', *, *, #25431, .F. ) ;
#22474=CARTESIAN_POINT ( 'NONE',  ( -25.47847050916410439, -26.57182937991348481, -1.500000000000001332 ) ) ;
#22477=EDGE_CURVE ( 'NONE', #11031, #7019, #27248, .T. ) ;
#22502=DIRECTION ( 'NONE',  ( -0.000000000000000000, 0.000000000000000000, 1.000000000000000000 ) ) ;
#22513=CARTESIAN_POINT ( 'NONE',  ( 2.552544031601107211, 42.49999999998228617, -1.500000000000000000 ) ) ;
#22522=CARTESIAN_POINT ( 'NONE',  ( 32.74775157612609178, -27.21557300919356948, -19.50000000000000355 ) ) ;
#22540=VECTOR ( 'NONE', #6088, 1000.000000000000000 ) ;
#22544=CARTESIAN_POINT ( 'NONE',  ( -40.05520497409654013, 7.028746409781321702, -16.50000000000000000 ) ) ;
#22548=ORIENTED_EDGE ( 'NONE', *, *, #27123, .F. ) ;
#22552=VERTEX_POINT ( 'NONE', #1966 ) ;
#22554=CARTESIAN_POINT ( 'NONE',  ( 39.83602371821015709, 11.57901747687536265, -19.50000000000000355 ) ) ;
#22584=VERTEX_POINT ( 'NONE', #18813 ) ;
#22586=AXIS2_PLACEMENT_3D ( 'NONE', #14347, #12328, #26364 ) ;
#22627=EDGE_LOOP ( 'NONE', ( #1621, #3380, #21526, #27706 ) ) ;
#22631=( NAMED_UNIT ( * ) SI_UNIT ( $, .STERADIAN. ) SOLID_ANGLE_UNIT ( ) );
#22661=CARTESIAN_POINT ( 'NONE',  ( 5.374868878255610660, 44.10336124695606230, -19.50000000000000355 ) ) ;
#22666=CARTESIAN_POINT ( 'NONE',  ( 34.07766914598172292, -21.40380666527112652, -1.500000000000000000 ) ) ;
#22671=CARTESIAN_POINT ( 'NONE',  ( 5.105024945674004222, 42.22604126506330857, -1.500000000000000000 ) ) ;
#22676=ORIENTED_EDGE ( 'NONE', *, *, #29297, .T. ) ;
#22698=DIRECTION ( 'NONE',  ( -1.000000000000000000, 0.000000000000000000, 0.000000000000000000 ) ) ;
#22702=CARTESIAN_POINT ( 'NONE',  ( -40.89187623478217404, -5.790488632116337797, -19.50000000000000355 ) ) ;
#22707=EDGE_CURVE ( 'NONE', #22552, #26111, #14109, .T. ) ;
#22738=DIRECTION ( 'NONE',  ( 0.06975647374412530244, 0.000000000000000000, 0.9975640502598241977 ) ) ;
#22739=AXIS2_PLACEMENT_3D ( 'NONE', #1310, #24393, #19711 ) ;
#22760=ORIENTED_EDGE ( 'NONE', *, *, #19679, .F. ) ;
#22765=ORIENTED_EDGE ( 'NONE', *, *, #4701, .F. ) ;
#22790=CARTESIAN_POINT ( 'NONE',  ( -25.64627119138473432, 23.40052582045089480, -16.50000000000000000 ) ) ;
#22815=CARTESIAN_POINT ( 'NONE',  ( -23.20738078402527549, -23.09073189384302793, -16.50001200000000523 ) ) ;
#22826=CARTESIAN_POINT ( 'NONE',  ( 0.000000000000000000, 44.39187623478217404, -19.50000000000000355 ) ) ;
#22831=CARTESIAN_POINT ( 'NONE',  ( -35.76344986165604212, -22.29344514668547461, -19.50000000000000355 ) ) ;
#22837=CARTESIAN_POINT ( 'NONE',  ( 39.00000000000000000, 5.563236990218597633, -1.500000000000000000 ) ) ;
#22840=B_SPLINE_SURFACE_WITH_KNOTS ( 'NONE', 1, 3, ( 
 ( #1763, #18757, #23270, #20926, #4408, #4556, #13924, #14060, #30005, #27661, #25322, #29036, #4709, #11899, #30755, #18918, #12194, #19372, #28892, #9544, #14680, #12358, #9857, #175, #2836, #32, #17024, #26075, #9695, #14209, #21861, #5329, #9401, #14838, #28426, #7050, #26548, #12046, #496, #7526, #2532, #23723 ),
 ( #4865, #2214, #16716, #5175, #26227, #21224, #2371, #10016, #26396, #21392, #19204, #16557, #19057, #28574, #14381, #7677, #17177, #7203, #21540, #23888, #28733, #26697, #24183, #7369, #11731, #16878, #5021, #14534, #24032, #2679, #21692, #333, #10627, #12518, #17650, #3148, #1115, #10315, #24971, #29188, #24658, #792 ) ),
 .UNSPECIFIED., .F., .T., .F.,
 ( 2, 2 ),
 ( 4, 2, 2, 2, 2, 2, 2, 2, 2, 2, 2, 2, 2, 2, 2, 2, 2, 2, 2, 2, 4 ),
 ( 0.000000000000000000, 1.000000000000000000 ),
 ( 0.000000000000000000, 0.1963495408493620697, 0.3926990816987241395, 0.7853981633974482790, 1.178097245096172418, 1.570796326794896558, 1.963495408493620697, 2.356194490192344837, 2.748893571891068976, 2.945243112740430824, 3.141592653589793116, 3.337942194439155408, 3.534291735288517255, 3.926990816987241395, 4.319689898685965090, 4.712388980384689674, 5.105088062083414258, 5.497787143782137953, 5.890486225480861648, 6.086835766330223940, 6.283185307179586232 ),
 .UNSPECIFIED. ) ;
#22866=CARTESIAN_POINT ( 'NONE',  ( -35.76344986165608475, 22.29344514668535027, -19.50000000000000355 ) ) ;
#22870=CARTESIAN_POINT ( 'NONE',  ( 23.05654803568420874, -35.38768970123555135, -9.833278305091164739 ) ) ;
#22888=AXIS2_PLACEMENT_3D ( 'NONE', #11672, #9179, #18692 ) ;
#22897=DIRECTION ( 'NONE',  ( -0.9975640502598243087, 0.000000000000000000, 0.06975647374412531632 ) ) ;
#22900=ORIENTED_EDGE ( 'NONE', *, *, #7113, .T. ) ;
#22915=DIRECTION ( 'NONE',  ( -0.000000000000000000, -0.000000000000000000, -1.000000000000000000 ) ) ;
#22918=ORIENTED_EDGE ( 'NONE', *, *, #14549, .T. ) ;
#22924=EDGE_CURVE ( 'NONE', #4162, #21118, #4378, .T. ) ;
#22927=CARTESIAN_POINT ( 'NONE',  ( -39.52380524535562500, 7.028748154183637631, -6.500000000000000888 ) ) ;
#22949=DIRECTION ( 'NONE',  ( -1.000000000000000000, 0.000000000000000000, 0.000000000000000000 ) ) ;
#22972=CARTESIAN_POINT ( 'NONE',  ( -37.98493438988125348, -11.12428508575252728, -1.500000000000000000 ) ) ;
#22977=CARTESIAN_POINT ( 'NONE',  ( -25.19442432475839055, 35.44676296258369064, -19.50000000000000355 ) ) ;
#22983=CARTESIAN_POINT ( 'NONE',  ( -13.22505861668184046, -42.10773672057003125, -19.50000000000000355 ) ) ;
#23003=CARTESIAN_POINT ( 'NONE',  ( -32.24119420145671455, 26.76047160551536663, -16.50000600000000262 ) ) ;
#23004=AXIS2_PLACEMENT_3D ( 'NONE', #15415, #22437, #16720 ) ;
#23010=CARTESIAN_POINT ( 'NONE',  ( 20.65888525914375862, -38.75220717792901581, -19.50000000000000355 ) ) ;
#23019=DIRECTION ( 'NONE',  ( -1.000000000000000000, 0.000000000000000000, 0.000000000000000000 ) ) ;
#23020=CARTESIAN_POINT ( 'NONE',  ( -5.206534544686763688, -43.71581230463343104, -16.50000000000000000 ) ) ;
#23030=CARTESIAN_POINT ( 'NONE',  ( -39.52380524535903561, -7.028748154198949827, -11.49999999999999645 ) ) ;
#23038=CARTESIAN_POINT ( 'NONE',  ( 33.16313691975489064, 0.000000000000000000, -1.500000000000000000 ) ) ;
#23056=EDGE_CURVE ( 'NONE', #5977, #15053, #13438, .T. ) ;
#23070=EDGE_CURVE ( 'NONE', #13268, #18557, #1970, .T. ) ;
#23101=VERTEX_POINT ( 'NONE', #18892 ) ;
#23129=CARTESIAN_POINT ( 'NONE',  ( -19.64114023396061981, 37.13592150528867109, -1.500000000000000000 ) ) ;
#23135=CARTESIAN_POINT ( 'NONE',  ( -35.76344986165608475, 22.29344514668535027, -19.50000000000000355 ) ) ;
#23145=EDGE_CURVE ( 'NONE', #26358, #8889, #22138, .T. ) ;
#23152=CARTESIAN_POINT ( 'NONE',  ( 31.29501345865701012, -26.27841684422097401, -6.499999999999999112 ) ) ;
#23162=CARTESIAN_POINT ( 'NONE',  ( 34.07766914600081520, 21.40380666527109810, -1.500000000000000000 ) ) ;
#23169=DIRECTION ( 'NONE',  ( 1.000000000000000000, -0.000000000000000000, 0.000000000000000000 ) ) ;
#23180=EDGE_CURVE ( 'NONE', #29503, #24153, #22150, .T. ) ;
#23182=CARTESIAN_POINT ( 'NONE',  ( -25.47847050916410439, -26.57182937991348481, 26.54355021145563143 ) ) ;
#23199=VECTOR ( 'NONE', #16523, 1000.000000000000000 ) ;
#23210=CARTESIAN_POINT ( 'NONE',  ( -26.41394434536923441, 32.09691347257119531, -6.500000000000000888 ) ) ;
#23239=CARTESIAN_POINT ( 'NONE',  ( 24.03057240117691862, 26.57182937991349903, -6.499999999999999112 ) ) ;
#23241=VECTOR ( 'NONE', #6370, 1000.000000000000000 ) ;
#23268=AXIS2_PLACEMENT_3D ( 'NONE', #18579, #8749, #16080 ) ;
#23270=CARTESIAN_POINT ( 'NONE',  ( 5.374868878255610660, 44.10336124695606230, -19.50000000000000355 ) ) ;
#23276=CARTESIAN_POINT ( 'NONE',  ( -19.64114023396299302, -37.13592150529018454, -1.500000000000000000 ) ) ;
#23325=CARTESIAN_POINT ( 'NONE',  ( -34.07766914599911701, 21.40380666528009002, -1.500000000000000000 ) ) ;
#23348=B_SPLINE_CURVE_WITH_KNOTS ( 'NONE', 3,
 ( #11326, #30635, #29778, #11478 ),
 .UNSPECIFIED., .F., .F.,
 ( 4, 4 ),
 ( 0.000000000000000000, 0.005028157979160071712 ),
 .UNSPECIFIED. ) ;
#23364=ADVANCED_FACE ( 'NONE', ( #30540 ), #4504, .T. ) ;
#23376=CARTESIAN_POINT ( 'NONE',  ( -29.15452456067305675, 29.11038375075762730, -6.500000000000000888 ) ) ;
#23378=ORIENTED_EDGE ( 'NONE', *, *, #23471, .F. ) ;
#23395=CARTESIAN_POINT ( 'NONE',  ( -12.56641067637752229, 40.32935944495016400, -1.500000000000009992 ) ) ;
#23397=CARTESIAN_POINT ( 'NONE',  ( 24.03057240117691862, -26.57182937991349903, -6.500000000000000888 ) ) ;
#23429=ORIENTED_EDGE ( 'NONE', *, *, #27289, .T. ) ;
#23437=CARTESIAN_POINT ( 'NONE',  ( -39.52380524535562500, 7.028748154183637631, -6.500000000000000888 ) ) ;
#23457=CARTESIAN_POINT ( 'NONE',  ( 30.26724724045159931, -27.72993536917819313, -6.500000000000000000 ) ) ;
#23471=EDGE_CURVE ( 'NONE', #11174, #6254, #2076, .T. ) ;
#23493=CARTESIAN_POINT ( 'NONE',  ( 6.780059429077784472, -43.46078076613360253, -16.50000000000000000 ) ) ;
#23510=ORIENTED_EDGE ( 'NONE', *, *, #10730, .F. ) ;
#23538=ORIENTED_EDGE ( 'NONE', *, *, #13051, .F. ) ;
#23542=DIRECTION ( 'NONE',  ( 1.000000000000000000, 0.000000000000000000, 0.000000000000000000 ) ) ;
#23566=VERTEX_POINT ( 'NONE', #20647 ) ;
#23577=CARTESIAN_POINT ( 'NONE',  ( -34.07766914599911701, 21.40380666528009002, -1.500000000000000000 ) ) ;
#23578=CARTESIAN_POINT ( 'NONE',  ( 32.74775157611827581, 27.21557300921217859, -19.50000000000000355 ) ) ;
#23579=ORIENTED_EDGE ( 'NONE', *, *, #4218, .T. ) ;
#23581=CARTESIAN_POINT ( 'NONE',  ( -5.105024945673440229, 42.22604126506271172, -1.500000000000000000 ) ) ;
#23585=DIRECTION ( 'NONE',  ( -0.5503133621338230919, 0.8349582046168344540, 0.000000000000000000 ) ) ;
#23586=CARTESIAN_POINT ( 'NONE',  ( -19.64114023396061981, 37.13592150528867109, -1.500000000000000000 ) ) ;
#23589=ORIENTED_EDGE ( 'NONE', *, *, #29903, .T. ) ;
#23599=CARTESIAN_POINT ( 'NONE',  ( -1.096289798481170570E-10, -7.028748153765593365, -16.50000000000000000 ) ) ;
#23616=CARTESIAN_POINT ( 'NONE',  ( -2.552544031601109875, 42.50000000001772094, -1.500000000000000000 ) ) ;
#23617=CARTESIAN_POINT ( 'NONE',  ( -26.80246859415415273, -7.028748154183645624, -1.499999999999999556 ) ) ;
#23626=CARTESIAN_POINT ( 'NONE',  ( -13.28078564537778838, -41.66453699854426418, -16.49999999999999289 ) ) ;
#23655=B_SPLINE_CURVE_WITH_KNOTS ( 'NONE', 3,
 ( #7590, #28497, #19437, #28954, #21924, #10074, #7127, #11968, #14277, #16639 ),
 .UNSPECIFIED., .F., .F.,
 ( 4, 2, 2, 2, 4 ),
 ( 0.000000000000000000, 0.007809271317857106529, 0.01561854263571419571, 0.03123708527142839142, 0.03978722987217712947 ),
 .UNSPECIFIED. ) ;
#23667=ADVANCED_FACE ( 'NONE', ( #24052 ), #2698, .F. ) ;
#23676=CARTESIAN_POINT ( 'NONE',  ( 20.46975788395958418, -26.57181885929544407, -16.50000600000000262 ) ) ;
#23677=CARTESIAN_POINT ( 'NONE',  ( 5.204170427930421283E-15, -44.07656352898514740, -16.50000000000000000 ) ) ;
#23723=CARTESIAN_POINT ( 'NONE',  ( 0.000000000000000000, 44.39187623478217404, -19.50000000000000355 ) ) ;
#23731=AXIS2_PLACEMENT_3D ( 'NONE', #26116, #5220, #78 ) ;
#23734=CARTESIAN_POINT ( 'NONE',  ( -12.56641067637752229, 40.32935944495016400, -1.500000000000000000 ) ) ;
#23741=CARTESIAN_POINT ( 'NONE',  ( 5.105024945673418912, -42.22604126506271882, -1.500000000000000000 ) ) ;
#23770=CARTESIAN_POINT ( 'NONE',  ( -26.80246859415415273, -7.028748154183637631, -1.499999999999999556 ) ) ;
#23774=VECTOR ( 'NONE', #16784, 1000.000000000000000 ) ;
#23776=CARTESIAN_POINT ( 'NONE',  ( -34.07766914599908148, -21.40380666528021081, -1.500000000000000000 ) ) ;
#23791=CARTESIAN_POINT ( 'NONE',  ( 0.000000000000000000, 0.000000000000000000, -1.500000000000001332 ) ) ;
#23796=CARTESIAN_POINT ( 'NONE',  ( 4.147066042697082011, 43.86011627092103993, -16.49999999999999645 ) ) ;
#23820=EDGE_CURVE ( 'NONE', #4151, #2298, #16579, .T. ) ;
#23827=CARTESIAN_POINT ( 'NONE',  ( -33.16313691975489064, 0.000000000000000000, -1.500000000000000000 ) ) ;
#23829=CARTESIAN_POINT ( 'NONE',  ( -32.81350286003733885, -7.028748154183637631, -6.500000000000000888 ) ) ;
#23830=EDGE_LOOP ( 'NONE', ( #28453, #29641, #26045, #19226 ) ) ;
#23836=VERTEX_POINT ( 'NONE', #10491 ) ;
#23837=EDGE_CURVE ( 'NONE', #30377, #3296, #19495, .T. ) ;
#23838=CARTESIAN_POINT ( 'NONE',  ( 24.03057240117690441, -26.57182937991349903, -1.500000000000001332 ) ) ;
#23849=ORIENTED_EDGE ( 'NONE', *, *, #6510, .F. ) ;
#23853=CARTESIAN_POINT ( 'NONE',  ( 25.10662277403243436, -23.12558862862892184, -16.50001200000000168 ) ) ;
#23859=AXIS2_PLACEMENT_3D ( 'NONE', #6949, #9280, #6783 ) ;
#23879=CARTESIAN_POINT ( 'NONE',  ( -39.87350638640939593, 4.706224724266459880, -11.49999999999999645 ) ) ;
#23882=CARTESIAN_POINT ( 'NONE',  ( -7.500000000000000000, 0.000000000000000000, -16.50000000000000000 ) ) ;
#23888=CARTESIAN_POINT ( 'NONE',  ( 5.105024945673418912, -42.22604126506271882, -1.500000000000000000 ) ) ;
#23893=ADVANCED_FACE ( 'NONE', ( #5660 ), #15157, .T. ) ;
#23898=CARTESIAN_POINT ( 'NONE',  ( 40.89187623478217404, -5.790488632116400858, -19.50000000000000355 ) ) ;
#23930=DIRECTION ( 'NONE',  ( -1.000000000000000000, 0.000000000000000000, 0.000000000000000000 ) ) ;
#23947=CARTESIAN_POINT ( 'NONE',  ( -18.02176112063609636, -39.50256893433222416, -16.50000000000000000 ) ) ;
#23949=ORIENTED_EDGE ( 'NONE', *, *, #18931, .F. ) ;
#23953=AXIS2_PLACEMENT_3D ( 'NONE', #24899, #6023, #15843 ) ;
#23954=CARTESIAN_POINT ( 'NONE',  ( 17.08170687911586327, 39.99681618153512375, -16.50000000000000711 ) ) ;
#23965=CARTESIAN_POINT ( 'NONE',  ( 22.58267429318971864, 26.57182937991349903, -6.499999999999999112 ) ) ;
#23973=CARTESIAN_POINT ( 'NONE',  ( 31.29501345865701012, -26.27841684422097401, -6.499999999999999112 ) ) ;
#23998=CARTESIAN_POINT ( 'NONE',  ( 39.87350638640253919, -4.706224724400470016, -11.49999999999999645 ) ) ;
#24008=CARTESIAN_POINT ( 'NONE',  ( -32.24119442679361214, -26.76047168400493703, -16.50000600000000262 ) ) ;
#24012=CARTESIAN_POINT ( 'NONE',  ( -33.46566279634613039, 23.92259740141228264, -11.49999999999999645 ) ) ;
#24013=EDGE_CURVE ( 'NONE', #7851, #26358, #8356, .T. ) ;
#24032=CARTESIAN_POINT ( 'NONE',  ( -34.07766914599908148, -21.40380666528021081, -1.500000000000000000 ) ) ;
#24040=CARTESIAN_POINT ( 'NONE',  ( -5.105024945675580739, -42.22604126506273303, -1.500000000000000000 ) ) ;
#24049=ORIENTED_EDGE ( 'NONE', *, *, #23820, .F. ) ;
#24052=FACE_OUTER_BOUND ( 'NONE', #1569, .T. ) ;
#24054=ORIENTED_EDGE ( 'NONE', *, *, #27092, .T. ) ;
#24066=ORIENTED_EDGE ( 'NONE', *, *, #15116, .F. ) ;
#24070=DIRECTION ( 'NONE',  ( -0.000000000000000000, -0.000000000000000000, -1.000000000000000000 ) ) ;
#24071=CARTESIAN_POINT ( 'NONE',  ( 8.065487902651284458, -43.19822004875265264, -16.49999999999999645 ) ) ;
#24075=CIRCLE ( 'NONE', #162, 3.559164065751841743 ) ;
#24078=DIRECTION ( 'NONE',  ( 1.000000000000000000, 0.000000000000000000, 0.000000000000000000 ) ) ;
#24108=VERTEX_POINT ( 'NONE', #2815 ) ;
#24117=PLANE ( 'NONE',  #5421 ) ;
#24131=EDGE_CURVE ( 'NONE', #3032, #14088, #14192, .T. ) ;
#24153=VERTEX_POINT ( 'NONE', #24008 ) ;
#24176=CARTESIAN_POINT ( 'NONE',  ( -22.58267429318971864, 26.57182937991348481, -6.499999999999999112 ) ) ;
#24183=CARTESIAN_POINT ( 'NONE',  ( -5.105024945675580739, -42.22604126506273303, -1.500000000000000000 ) ) ;
#24191=CARTESIAN_POINT ( 'NONE',  ( -2.687479362164884034, -44.39187623478217404, -19.50000000000000355 ) ) ;
#24205=ORIENTED_EDGE ( 'NONE', *, *, #22148, .F. ) ;
#24212=EDGE_CURVE ( 'NONE', #5571, #30328, #17946, .T. ) ;
#24217=CARTESIAN_POINT ( 'NONE',  ( -22.21046885174908425, 23.49239644259613158, -16.50001200000000168 ) ) ;
#24242=ADVANCED_FACE ( 'NONE', ( #10931 ), #27765, .F. ) ;
#24257=AXIS2_PLACEMENT_3D ( 'NONE', #21436, #7564, #23930 ) ;
#24266=CARTESIAN_POINT ( 'NONE',  ( 14.24118286736276850, 41.28857907310604958, -16.50000000000000355 ) ) ;
#24280=EDGE_CURVE ( 'NONE', #15207, #26111, #9183, .T. ) ;
#24286=EDGE_CURVE ( 'NONE', #4162, #3753, #4345, .T. ) ;
#24303=ORIENTED_EDGE ( 'NONE', *, *, #23820, .T. ) ;
#24334=FACE_OUTER_BOUND ( 'NONE', #12304, .T. ) ;
#24360=CARTESIAN_POINT ( 'NONE',  ( -20.65888525914099105, 38.75220717792564784, -19.50000000000000355 ) ) ;
#24388=ORIENTED_EDGE ( 'NONE', *, *, #9196, .F. ) ;
#24389=VECTOR ( 'NONE', #28937, 1000.000000000000000 ) ;
#24393=DIRECTION ( 'NONE',  ( 0.8349582046168341209, -0.5503133621338236470, 0.000000000000000000 ) ) ;
#24415=CARTESIAN_POINT ( 'NONE',  ( 40.05520497557499482, 7.028746409576331011, -16.50000000000000000 ) ) ;
#24429=ADVANCED_FACE ( 'NONE', ( #19466 ), #16361, .F. ) ;
#24430=DIRECTION ( 'NONE',  ( -1.000000000000000000, 0.000000000000000000, 0.000000000000000000 ) ) ;
#24438=CARTESIAN_POINT ( 'NONE',  ( -24.03057240117691862, 26.57182937991348481, -6.499999999999999112 ) ) ;
#24446=VERTEX_POINT ( 'NONE', #21645 ) ;
#24453=ORIENTED_EDGE ( 'NONE', *, *, #23056, .F. ) ;
#24469=VECTOR ( 'NONE', #18801, 1000.000000000000000 ) ;
#24479=CARTESIAN_POINT ( 'NONE',  ( -31.29501345865529061, -26.27841684422010360, -6.500000000000000888 ) ) ;
#24505=ORIENTED_EDGE ( 'NONE', *, *, #4666, .F. ) ;
#24511=CARTESIAN_POINT ( 'NONE',  ( -39.83602371821029919, -11.57901747687044924, -19.50000000000000355 ) ) ;
#24534=CARTESIAN_POINT ( 'NONE',  ( 25.64627119138473432, 23.40052582045089480, -16.50000000000000000 ) ) ;
#24538=ORIENTED_EDGE ( 'NONE', *, *, #23056, .T. ) ;
#24545=CARTESIAN_POINT ( 'NONE',  ( -40.89187623478217404, -5.790488632116337797, -19.50000000000000355 ) ) ;
#24553=SHAPE_DEFINITION_REPRESENTATION ( #18886, #16871 ) ;
#24557=ORIENTED_EDGE ( 'NONE', *, *, #19679, .T. ) ;
#24574=CARTESIAN_POINT ( 'NONE',  ( -40.35746994301763380, -4.708323662206837845, -16.50000000000000355 ) ) ;
#24597=EDGE_CURVE ( 'NONE', #19456, #19866, #11685, .T. ) ;
#24648=FACE_OUTER_BOUND ( 'NONE', #29015, .T. ) ;
#24658=CARTESIAN_POINT ( 'NONE',  ( -2.552544031601109875, 42.50000000001772094, -1.500000000000000000 ) ) ;
#24697=CARTESIAN_POINT ( 'NONE',  ( 23.96732207937828463, 33.98584080152456011, -1.500000000000000000 ) ) ;
#24704=CARTESIAN_POINT ( 'NONE',  ( -40.89187623478217404, 5.790488632116478129, -19.50000000000000355 ) ) ;
#24721=CARTESIAN_POINT ( 'NONE',  ( -25.64627119138473432, -23.40052582045089480, -16.50000000000000000 ) ) ;
#24732=CARTESIAN_POINT ( 'NONE',  ( -25.47847050916411504, 26.57182937991348481, -1.500000000000001332 ) ) ;
#24733=STYLED_ITEM('',(#30893),#2654);
#24737=CARTESIAN_POINT ( 'NONE',  ( -25.23756106473024730, -11.43858098102957577, -11.49999999999999645 ) ) ;
#24752=AXIS2_PLACEMENT_3D ( 'NONE', #645, #5330, #5795 ) ;
#24757=CARTESIAN_POINT ( 'NONE',  ( 39.87350638640939593, 4.706224724266460768, -11.49999999999999645 ) ) ;
#24764=DIRECTION ( 'NONE',  ( 0.06975647374412530244, -0.000000000000000000, -0.9975640502598241977 ) ) ;
#24769=CARTESIAN_POINT ( 'NONE',  ( -12.33859880789482233, -8.132258305203423632, -16.50000000000000000 ) ) ;
#24810=CARTESIAN_POINT ( 'NONE',  ( -39.87350638640939593, 4.706224724266459880, -6.500000000000000888 ) ) ;
#24812=VECTOR ( 'NONE', #19650, 1000.000000000000000 ) ;
#24838=EDGE_CURVE ( 'NONE', #13692, #13938, #3108, .T. ) ;
#24850=EDGE_LOOP ( 'NONE', ( #15658, #20917 ) ) ;
#24860=CARTESIAN_POINT ( 'NONE',  ( 20.71335220384823117, -27.86167394782616213, -16.50000000000000000 ) ) ;
#24870=CARTESIAN_POINT ( 'NONE',  ( -39.83602371821029919, -11.57901747687044924, -19.50000000000000355 ) ) ;
#24876=CARTESIAN_POINT ( 'NONE',  ( -19.64114023396299302, -37.13592150529018454, -1.500000000000000000 ) ) ;
#24879=EDGE_LOOP ( 'NONE', ( #5532, #22765, #27189, #16787 ) ) ;
#24887=EDGE_LOOP ( 'NONE', ( #5718, #24303, #24954, #26452, #24557 ) ) ;
#24899=CARTESIAN_POINT ( 'NONE',  ( 24.03057240117691862, 26.57182937991349903, -16.50000000000000000 ) ) ;
#24906=EDGE_LOOP ( 'NONE', ( #10579, #6970, #8892, #4760 ) ) ;
#24908=CARTESIAN_POINT ( 'NONE',  ( 10.64374042650304020, -42.96126232887725394, -19.50000000000000355 ) ) ;
#24954=ORIENTED_EDGE ( 'NONE', *, *, #4701, .T. ) ;
#24963=CARTESIAN_POINT ( 'NONE',  ( -20.71335220384823117, 27.86167394782616213, -6.500000000000000888 ) ) ;
#24964=CARTESIAN_POINT ( 'NONE',  ( -40.05104235265675783, 2.353288714454549790, -6.500000000000000888 ) ) ;
#24971=CARTESIAN_POINT ( 'NONE',  ( -10.11202017158466759, 41.14070756921185534, -1.500000000000000000 ) ) ;
#24982=ORIENTED_EDGE ( 'NONE', *, *, #8795, .F. ) ;
#24997=CARTESIAN_POINT ( 'NONE',  ( -35.78163722268750746, 27.43648963448195133, -11.49999999999999645 ) ) ;
#25002=LINE ( 'NONE', #10979, #19735 ) ;
#25011=CARTESIAN_POINT ( 'NONE',  ( 7.500000000000000000, 9.184850993605147944E-16, 63.50000000000000000 ) ) ;
#25015=CARTESIAN_POINT ( 'NONE',  ( 5.374868878254059013, -44.10336124695543703, -19.50000000000000355 ) ) ;
#25020=CARTESIAN_POINT ( 'NONE',  ( -25.19442432475474902, -35.44676296258422354, -19.50000000000000355 ) ) ;
#25024=CARTESIAN_POINT ( 'NONE',  ( 19.64114023396890829, 37.13592150528549496, -1.500000000000000000 ) ) ;
#25045=CARTESIAN_POINT ( 'NONE',  ( -40.57621058660762259, -1.187786509009159941, -16.50000000000000000 ) ) ;
#25046=FACE_OUTER_BOUND ( 'NONE', #8768, .T. ) ;
#25058=ORIENTED_EDGE ( 'NONE', *, *, #4641, .F. ) ;
#25060=DIRECTION ( 'NONE',  ( -1.000000000000000000, 0.000000000000000000, 0.000000000000000000 ) ) ;
#25062=CIRCLE ( 'NONE', #26060, 3.559164065751841743 ) ;
#25073=ORIENTED_EDGE ( 'NONE', *, *, #7930, .F. ) ;
#25082=AXIS2_PLACEMENT_3D ( 'NONE', #13011, #22502, #8026 ) ;
#25115=CARTESIAN_POINT ( 'NONE',  ( -25.47847050916410439, -26.57182937991348481, -6.499999999999999112 ) ) ;
#25132=DIRECTION ( 'NONE',  ( -0.8910248307962438385, 0.4539545692076743522, 0.000000000000000000 ) ) ;
#25150=CARTESIAN_POINT ( 'NONE',  ( -20.50469103882543109, -27.17502484134976015, -16.50001200000000523 ) ) ;
#25160=CARTESIAN_POINT ( 'NONE',  ( 20.65888525914559892, 38.75220717792412728, -19.50000000000000355 ) ) ;
#25162=VERTEX_POINT ( 'NONE', #9937 ) ;
#25167=CARTESIAN_POINT ( 'NONE',  ( 2.687479362164894248, -44.39187623478217404, -19.50000000000000355 ) ) ;
#25172=CARTESIAN_POINT ( 'NONE',  ( 2.687479363073301819, 44.39187623479102740, -19.50000000000000355 ) ) ;
#25202=ORIENTED_EDGE ( 'NONE', *, *, #12657, .T. ) ;
#25205=CARTESIAN_POINT ( 'NONE',  ( 13.22505861668094340, 42.10773672057246841, -19.50000000000000355 ) ) ;
#25211=EDGE_CURVE ( 'NONE', #29282, #4972, #14984, .T. ) ;
#25223=DIRECTION ( 'NONE',  ( -1.000000000000000000, 0.000000000000000000, 0.000000000000000000 ) ) ;
#25224=ORIENTED_EDGE ( 'NONE', *, *, #19283, .T. ) ;
#25250=ORIENTED_EDGE ( 'NONE', *, *, #9154, .F. ) ;
#25266=AXIS2_PLACEMENT_3D ( 'NONE', #28230, #5140, #14651 ) ;
#25287=VERTEX_POINT ( 'NONE', #24732 ) ;
#25309=EDGE_LOOP ( 'NONE', ( #3001, #17970, #11259, #11485, #14989, #23949, #27630, #2752, #25250, #13593, #12225, #28407, #1246, #22676, #6249, #23849, #27930, #28707 ) ) ;
#25322=CARTESIAN_POINT ( 'NONE',  ( 40.89187623478217404, 5.790488632116406187, -19.50000000000000355 ) ) ;
#25326=CARTESIAN_POINT ( 'NONE',  ( -10.11202017158466759, 41.14070756921185534, -1.500000000000000000 ) ) ;
#25332=CARTESIAN_POINT ( 'NONE',  ( -13.22505861668184046, -42.10773672057003125, -19.50000000000000355 ) ) ;
#25337=CARTESIAN_POINT ( 'NONE',  ( 5.374868878254059013, -44.10336124695543703, -19.50000000000000355 ) ) ;
#25353=B_SPLINE_CURVE_WITH_KNOTS ( 'NONE', 3,
 ( #7375, #14065, #25931, #17029, #26233 ),
 .UNSPECIFIED., .F., .F.,
 ( 4, 1, 4 ),
 ( 0.3464918507984035556, 0.3518176900574713217, 0.3571435293165390878 ),
 .UNSPECIFIED. ) ;
#25377=CARTESIAN_POINT ( 'NONE',  ( 26.80246859415415273, -7.028748154183637631, -1.499999999999999556 ) ) ;
#25382=B_SPLINE_CURVE_WITH_KNOTS ( 'NONE', 3,
 ( #23152, #23457, #25968, #18188, #1654, #11322 ),
 .UNSPECIFIED., .F., .F.,
 ( 4, 2, 4 ),
 ( 0.001794032523744855520, 0.007046146517949118150, 0.01388807892444184240 ),
 .UNSPECIFIED. ) ;
#25384=DIRECTION ( 'NONE',  ( 0.000000000000000000, 0.000000000000000000, -1.000000000000000000 ) ) ;
#25385=CARTESIAN_POINT ( 'NONE',  ( -3.653991135135629342, -43.89827854335435120, -16.50000000000000355 ) ) ;
#25391=ADVANCED_FACE ( 'NONE', ( #12905 ), #11325, .T. ) ;
#25397=EDGE_CURVE ( 'NONE', #24446, #28753, #30343, .T. ) ;
#25402=LINE ( 'NONE', #18394, #8070 ) ;
#25431=EDGE_CURVE ( 'NONE', #13626, #26229, #1958, .T. ) ;
#25432=CIRCLE ( 'NONE', #3952, 1.447898107987198646 ) ;
#25460=EDGE_CURVE ( 'NONE', #12213, #14363, #2099, .T. ) ;
#25464=ORIENTED_EDGE ( 'NONE', *, *, #13501, .T. ) ;
#25488=CARTESIAN_POINT ( 'NONE',  ( -2.552544030762004645, -42.50000000000000000, -1.500000000000000000 ) ) ;
#25499=CARTESIAN_POINT ( 'NONE',  ( -25.19442432475839055, 35.44676296258369064, -19.50000000000000355 ) ) ;
#25500=CARTESIAN_POINT ( 'NONE',  ( 20.71335220384823117, 27.86167394782616213, -6.500000000000000888 ) ) ;
#25503=AXIS2_PLACEMENT_3D ( 'NONE', #16492, #18993, #26009 ) ;
#25508=AXIS2_PLACEMENT_3D ( 'NONE', #19129, #11646, #9468 ) ;
#25522=DIRECTION ( 'NONE',  ( -0.000000000000000000, -0.000000000000000000, 1.000000000000000000 ) ) ;
#25525=CARTESIAN_POINT ( 'NONE',  ( 33.78553873773097393, 24.40792641592722134, -16.50000000000000000 ) ) ;
#25530=CARTESIAN_POINT ( 'NONE',  ( -32.82330813384598400, -22.94799032726886523, -1.500000000000000000 ) ) ;
#25533=LINE ( 'NONE', #4159, #12821 ) ;
#25546=CARTESIAN_POINT ( 'NONE',  ( 10.58893626534552190, -42.55607912659770165, -16.49999999999999645 ) ) ;
#25573=DIRECTION ( 'NONE',  ( -0.000000000000000000, -0.000000000000000000, -1.000000000000000000 ) ) ;
#25580=VERTEX_POINT ( 'NONE', #10972 ) ;
#25588=CARTESIAN_POINT ( 'NONE',  ( 24.73258466867332572, 33.64422401625767378, -6.500000000000000888 ) ) ;
#25621=CARTESIAN_POINT ( 'NONE',  ( -1.046997975306281248, 44.06280042554938348, -16.50000000000000355 ) ) ;
#25623=CARTESIAN_POINT ( 'NONE',  ( -23.11204207310937875, -35.56592875159903855, -11.49994540249954156 ) ) ;
#25626=CARTESIAN_POINT ( 'NONE',  ( -23.91679456219654298, -22.99653376284463491, -16.50001200000000168 ) ) ;
#25627=VECTOR ( 'NONE', #20074, 1000.000000000000000 ) ;
#25631=EDGE_CURVE ( 'NONE', #8392, #4264, #19449, .T. ) ;
#25638=CARTESIAN_POINT ( 'NONE',  ( -23.96732207938974213, -33.98584080153308662, -1.500000000000000000 ) ) ;
#25647=CARTESIAN_POINT ( 'NONE',  ( -39.00000000000000000, -5.563236990218529243, -1.500000000000000000 ) ) ;
#25659=LINE ( 'NONE', #4279, #21316 ) ;
#25674=CARTESIAN_POINT ( 'NONE',  ( 19.64114023396309960, -37.13592150529014191, -1.500000000000000000 ) ) ;
#25676=ORIENTED_EDGE ( 'NONE', *, *, #12657, .F. ) ;
#25683=CARTESIAN_POINT ( 'NONE',  ( -8.275208547106167600, -43.16521806348789880, -16.50000000000000000 ) ) ;
#25708=EDGE_LOOP ( 'NONE', ( #123, #17244, #4230, #24066 ) ) ;
#25741=CARTESIAN_POINT ( 'NONE',  ( 33.13218612630368654, -7.028748154183637631, -1.942616967526160643 ) ) ;
#25742=DIRECTION ( 'NONE',  ( -0.000000000000000000, 0.000000000000000000, -1.000000000000000000 ) ) ;
#25750=ORIENTED_EDGE ( 'NONE', *, *, #455, .F. ) ;
#25751=AXIS2_PLACEMENT_3D ( 'NONE', #25925, #17023, #7048 ) ;
#25760=CARTESIAN_POINT ( 'NONE',  ( -7.281713232848989747, 43.36492703356076817, -16.49999999999999645 ) ) ;
#25769=AXIS2_PLACEMENT_3D ( 'NONE', #2161, #9339, #8893 ) ;
#25776=ADVANCED_FACE ( 'NONE', ( #2824 ), #12346, .F. ) ;
#25848=CARTESIAN_POINT ( 'NONE',  ( 0.000000000000000000, 0.000000000000000000, -1.500000000000000000 ) ) ;
#25925=CARTESIAN_POINT ( 'NONE',  ( -24.03057240117690441, -26.57182937991348481, -1.500000000000001332 ) ) ;
#25928=ORIENTED_EDGE ( 'NONE', *, *, #29644, .T. ) ;
#25931=CARTESIAN_POINT ( 'NONE',  ( -33.03678701508917470, 25.60268426854908697, -16.50000000000000000 ) ) ;
#25933=CARTESIAN_POINT ( 'NONE',  ( 22.58267429318970443, -26.57182937991349903, -1.500000000000001332 ) ) ;
#25935=DIRECTION ( 'NONE',  ( -1.000000000000000000, 0.000000000000000000, 0.000000000000000000 ) ) ;
#25943=B_SPLINE_CURVE_WITH_KNOTS ( 'NONE', 3,
 ( #21307, #15876, #27892, #11649 ),
 .UNSPECIFIED., .F., .F.,
 ( 4, 4 ),
 ( 0.000000000000000000, 0.005028157979644255586 ),
 .UNSPECIFIED. ) ;
#25968=CARTESIAN_POINT ( 'NONE',  ( 29.15452456067750475, -29.11038375076027762, -6.500000000000000000 ) ) ;
#25978=CARTESIAN_POINT ( 'NONE',  ( -10.64374042650306862, 42.96126232887723972, -19.50000000000000355 ) ) ;
#26006=CARTESIAN_POINT ( 'NONE',  ( 23.17549888352340659, -36.17843697208695630, -16.49999999999999645 ) ) ;
#26009=DIRECTION ( 'NONE',  ( -1.000000000000000000, 0.000000000000000000, -0.000000000000000000 ) ) ;
#26014=EDGE_CURVE ( 'NONE', #16473, #27870, #8592, .T. ) ;
#26030=B_SPLINE_CURVE_WITH_KNOTS ( 'NONE', 3,
 ( #2837, #11901, #176, #19058 ),
 .UNSPECIFIED., .F., .F.,
 ( 4, 4 ),
 ( 0.000000000000000000, 0.005028157979644231300 ),
 .UNSPECIFIED. ) ;
#26037=CARTESIAN_POINT ( 'NONE',  ( 20.47140768548292655, -27.01178922547192585, -16.50001200000000168 ) ) ;
#26045=ORIENTED_EDGE ( 'NONE', *, *, #9196, .T. ) ;
#26048=CARTESIAN_POINT ( 'NONE',  ( 21.22112865003566640, -24.30434497425369855, -16.50001199999999812 ) ) ;
#26049=CARTESIAN_POINT ( 'NONE',  ( -40.05104235265675783, 2.353288714454549790, -11.49999999999999645 ) ) ;
#26060=AXIS2_PLACEMENT_3D ( 'NONE', #2721, #30220, #8865 ) ;
#26064=CARTESIAN_POINT ( 'NONE',  ( -19.96030473831224583, 38.37413104131353947, -16.50000000000000000 ) ) ;
#26065=VERTEX_POINT ( 'NONE', #19277 ) ;
#26072=ORIENTED_EDGE ( 'NONE', *, *, #14549, .F. ) ;
#26075=CARTESIAN_POINT ( 'NONE',  ( -32.74775157610760346, -27.21557300919352329, -19.50000000000000355 ) ) ;
#26091=LINE ( 'NONE', #4122, #14608 ) ;
#26108=CARTESIAN_POINT ( 'NONE',  ( 23.00100564343818021, 35.20929534198214128, -8.166629675737638649 ) ) ;
#26111=VERTEX_POINT ( 'NONE', #21458 ) ;
#26116=CARTESIAN_POINT ( 'NONE',  ( 24.03057240117691862, 26.57182937991349903, -6.500000000000000888 ) ) ;
#26123=CARTESIAN_POINT ( 'NONE',  ( -39.00000000000000000, 5.563236990218665134, -1.500000000000000000 ) ) ;
#26128=EDGE_CURVE ( 'NONE', #29372, #20109, #407, .T. ) ;
#26134=DIRECTION ( 'NONE',  ( 0.000000000000000000, -0.000000000000000000, 1.000000000000000000 ) ) ;
#26170=EDGE_LOOP ( 'NONE', ( #25750, #29635, #25464, #18562, #5055, #9635, #4298 ) ) ;
#26196=CARTESIAN_POINT ( 'NONE',  ( 22.68724997019158707, -23.22071843469717933, -16.50001200000000523 ) ) ;
#26222=CARTESIAN_POINT ( 'NONE',  ( -31.29501345865529061, -26.27841684422010360, -6.500000000000000888 ) ) ;
#26227=CARTESIAN_POINT ( 'NONE',  ( 12.56641067637329812, 40.32935944495179115, -1.500000000000000000 ) ) ;
#26228=CYLINDRICAL_SURFACE ( 'NONE', #28256, 27.70876437800068359 ) ;
#26229=VERTEX_POINT ( 'NONE', #1332 ) ;
#26233=CARTESIAN_POINT ( 'NONE',  ( -32.24119420145671455, 26.76047160551536663, -16.50000600000000262 ) ) ;
#26244=CARTESIAN_POINT ( 'NONE',  ( 12.56641067637628240, -40.32935944494942504, -1.500000000000000000 ) ) ;
#26259=ORIENTED_EDGE ( 'NONE', *, *, #1976, .T. ) ;
#26260=CARTESIAN_POINT ( 'NONE',  ( 29.55332031600731213, 27.89853503085377895, -1.500000000000003997 ) ) ;
#26274=CARTESIAN_POINT ( 'NONE',  ( 10.11202017158463917, -41.14070756921186955, -1.500000000000000000 ) ) ;
#26281=CARTESIAN_POINT ( 'NONE',  ( -13.22505861668333083, 42.10773672057167261, -19.50000000000000355 ) ) ;
#26294=CARTESIAN_POINT ( 'NONE',  ( -17.09865819214518368, -39.97652765376174955, -16.50000000000000355 ) ) ;
#26332=CARTESIAN_POINT ( 'NONE',  ( 31.76816150327698551, 26.51947378151753298, -11.49999299644477446 ) ) ;
#26358=VERTEX_POINT ( 'NONE', #3176 ) ;
#26364=DIRECTION ( 'NONE',  ( 1.000000000000000000, 0.000000000000000000, 0.000000000000000000 ) ) ;
#26396=CARTESIAN_POINT ( 'NONE',  ( 34.07766914600081520, 21.40380666527109810, -1.500000000000000000 ) ) ;
#26406=CARTESIAN_POINT ( 'NONE',  ( -23.96732207939035675, 33.98584080153585774, -1.500000000000000000 ) ) ;
#26407=ORIENTED_EDGE ( 'NONE', *, *, #4959, .T. ) ;
#26411=VERTEX_POINT ( 'NONE', #18295 ) ;
#26427=CARTESIAN_POINT ( 'NONE',  ( 19.64114023396890829, 37.13592150528549496, -1.500000000000003997 ) ) ;
#26428=CARTESIAN_POINT ( 'NONE',  ( 23.27838112219106392, 36.10018657900367600, -16.50000600000000262 ) ) ;
#26445=CARTESIAN_POINT ( 'NONE',  ( 40.89187623478217404, -5.790488632116400858, -19.50000000000000355 ) ) ;
#26452=ORIENTED_EDGE ( 'NONE', *, *, #27487, .T. ) ;
#26462=CARTESIAN_POINT ( 'NONE',  ( 8.264668169643783813, 43.16767620126012872, -16.50000000000000000 ) ) ;
#26512=CARTESIAN_POINT ( 'NONE',  ( -31.31394823341756251, 25.51108937476248428, -1.500000000000009992 ) ) ;
#26538=DIRECTION ( 'NONE',  ( -1.000000000000000000, 0.000000000000000000, 0.000000000000000000 ) ) ;
#26548=CARTESIAN_POINT ( 'NONE',  ( -20.65888525914099105, 38.75220717792564784, -19.50000000000000355 ) ) ;
#26557=CARTESIAN_POINT ( 'NONE',  ( -25.19442432475839055, 35.44676296258369064, -19.50000000000000355 ) ) ;
#26582=EDGE_CURVE ( 'NONE', #4264, #16453, #4469, .T. ) ;
#26585=CARTESIAN_POINT ( 'NONE',  ( -20.78475560873934569, 25.06838084537526612, -16.50001200000000168 ) ) ;
#26595=CARTESIAN_POINT ( 'NONE',  ( 39.52380524535562500, 7.028748154183637631, -11.49999999999999645 ) ) ;
#26602=CARTESIAN_POINT ( 'NONE',  ( 25.19442432474404470, 35.44676296256560022, -19.50000000000000355 ) ) ;
#26608=CARTESIAN_POINT ( 'NONE',  ( 7.500000000000000000, 9.184850993605147944E-16, -1.500000000000001332 ) ) ;
#26620=CARTESIAN_POINT ( 'NONE',  ( 9.785366065393095170, 42.77971715303853273, -16.49999999999999645 ) ) ;
#26624=DIRECTION ( 'NONE',  ( -1.000000000000000000, 0.000000000000000000, -0.000000000000000000 ) ) ;
#26627=CARTESIAN_POINT ( 'NONE',  ( 33.78553947564427773, -24.40792753551981775, -16.50000000000000000 ) ) ;
#26682=CARTESIAN_POINT ( 'NONE',  ( -33.67904612011425058, 24.24635139330486311, -14.83330431405463656 ) ) ;
#26697=CARTESIAN_POINT ( 'NONE',  ( -2.552544030762004645, -42.50000000000000000, -1.500000000000000000 ) ) ;
#26704=DIRECTION ( 'NONE',  ( -0.8349582046168341209, -0.5503133621338236470, 0.000000000000000000 ) ) ;
#26706=CARTESIAN_POINT ( 'NONE',  ( 12.56641067637628240, -40.32935944494942504, -1.500000000000000000 ) ) ;
#26716=CARTESIAN_POINT ( 'NONE',  ( 25.64627119138473432, 23.40052582045089480, -6.500000000000000888 ) ) ;
#26737=LINE ( 'NONE', #24860, #19600 ) ;
#26776=CARTESIAN_POINT ( 'NONE',  ( 21.79411701110929656, 37.18463376297794554, -16.49999999999999645 ) ) ;
#26791=ORIENTED_EDGE ( 'NONE', *, *, #4317, .T. ) ;
#26796=ORIENTED_EDGE ( 'NONE', *, *, #18925, .F. ) ;
#26812=ORIENTED_EDGE ( 'NONE', *, *, #27112, .T. ) ;
#26838=EDGE_CURVE ( 'NONE', #14649, #4182, #20126, .T. ) ;
#26873=CARTESIAN_POINT ( 'NONE',  ( 23.96732207938043402, -33.98584080152387088, -1.500000000000000000 ) ) ;
#26895=CARTESIAN_POINT ( 'NONE',  ( -22.85987860430571317, 23.19171692911513105, -16.50001200000000523 ) ) ;
#26912=EDGE_CURVE ( 'NONE', #30725, #22552, #30253, .T. ) ;
#26917=ORIENTED_EDGE ( 'NONE', *, *, #4642, .F. ) ;
#26919=AXIS2_PLACEMENT_3D ( 'NONE', #28555, #12025, #21518 ) ;
#26936=CARTESIAN_POINT ( 'NONE',  ( -33.78553954455730235, -24.40792764007751359, -16.50000000000000000 ) ) ;
#26952=VERTEX_POINT ( 'NONE', #24963 ) ;
#26958=CARTESIAN_POINT ( 'NONE',  ( 0.000000000000000000, 7.028748154183637631, -16.50000000000000000 ) ) ;
#26967=ORIENTED_EDGE ( 'NONE', *, *, #25431, .T. ) ;
#26986=CARTESIAN_POINT ( 'NONE',  ( 33.16313691975489064, -7.028748154183637631, -1.500000000000000000 ) ) ;
#27009=DIRECTION ( 'NONE',  ( -1.000000000000000000, 0.000000000000000000, 0.000000000000000000 ) ) ;
#27025=CARTESIAN_POINT ( 'NONE',  ( 34.07766914598172292, -21.40380666527112652, -1.500000000000000000 ) ) ;
#27044=CARTESIAN_POINT ( 'NONE',  ( -24.27860874716794726, 23.00333360197816290, -16.50001200000000168 ) ) ;
#27048=CARTESIAN_POINT ( 'NONE',  ( 24.03057240117691862, 26.57182937991349903, 26.54355021145563143 ) ) ;
#27056=CARTESIAN_POINT ( 'NONE',  ( 13.22505861668195237, -42.10773672056998862, -19.50000000000000355 ) ) ;
#27061=CARTESIAN_POINT ( 'NONE',  ( 13.22505861668094340, 42.10773672057246841, -19.50000000000000355 ) ) ;
#27069=B_SPLINE_SURFACE_WITH_KNOTS ( 'NONE', 1, 3, ( 
 ( #13680, #20526, #15852, #20070, #25205, #8383, #18198, #6033, #17900, #22554, #27414, #27872, #8544, #30047, #13528, #1208, #23010, #15383, #24908, #6496, #18046, #20674, #30197, #13214, #16006, #10560, #29589, #8223, #3544, #27561, #22702, #1357, #13373, #22866, #1516, #2109, #11630, #26281, #25978, #4608, #4296, #14108 ),
 ( #6791, #18969, #2258, #28329, #13825, #21122, #30804, #28477, #23162, #13972, #18510, #4463, #30641, #30354, #30494, #19109, #25674, #1964, #20830, #8995, #11779, #9453, #7105, #9135, #4754, #2428, #16614, #9288, #23776, #85, #28011, #26123, #14257, #23325, #11952, #4916, #6642, #21443, #28628, #21283, #23616, #18812 ) ),
 .UNSPECIFIED., .F., .T., .F.,
 ( 2, 2 ),
 ( 4, 2, 2, 2, 2, 2, 2, 2, 2, 2, 2, 2, 2, 2, 2, 2, 2, 2, 2, 2, 4 ),
 ( 0.000000000000000000, 1.000000000000000000 ),
 ( 0.000000000000000000, 0.1963495408493620697, 0.3926990816987241395, 0.7853981633974482790, 1.178097245096172418, 1.570796326794896558, 1.963495408493620697, 2.356194490192344837, 2.748893571891068976, 2.945243112740430824, 3.141592653589793116, 3.337942194439155408, 3.534291735288517255, 3.926990816987241395, 4.319689898685965090, 4.712388980384689674, 5.105088062083414258, 5.497787143782137953, 5.890486225480861648, 6.086835766330223940, 6.283185307179586232 ),
 .UNSPECIFIED. ) ;
#27072=ADVANCED_FACE ( 'NONE', ( #30855 ), #11687, .F. ) ;
#27078=EDGE_CURVE ( 'NONE', #5571, #13268, #30411, .T. ) ;
#27084=LINE ( 'NONE', #3217, #28704 ) ;
#27092=EDGE_CURVE ( 'NONE', #16156, #26411, #9345, .T. ) ;
#27103=ORIENTED_EDGE ( 'NONE', *, *, #20311, .T. ) ;
#27112=EDGE_CURVE ( 'NONE', #6853, #26065, #10598, .T. ) ;
#27113=CARTESIAN_POINT ( 'NONE',  ( 40.05104235265675783, -2.353288714521559744, -11.49999999999999645 ) ) ;
#27123=EDGE_CURVE ( 'NONE', #13970, #7038, #1869, .T. ) ;
#27136=DIRECTION ( 'NONE',  ( -0.000000000000000000, -0.000000000000000000, -1.000000000000000000 ) ) ;
#27170=ORIENTED_EDGE ( 'NONE', *, *, #15915, .T. ) ;
#27182=CYLINDRICAL_SURFACE ( 'NONE', #27869, 1.447898107987198646 ) ;
#27189=ORIENTED_EDGE ( 'NONE', *, *, #10099, .T. ) ;
#27198=DIRECTION ( 'NONE',  ( -1.000000000000000000, 0.000000000000000000, 0.000000000000000000 ) ) ;
#27204=CARTESIAN_POINT ( 'NONE',  ( 40.89187623478217404, 5.790488632116406187, -19.50000000000000355 ) ) ;
#27209=CARTESIAN_POINT ( 'NONE',  ( 5.105024945674004222, 42.22604126506330857, -1.500000000000000000 ) ) ;
#27215=CARTESIAN_POINT ( 'NONE',  ( 40.89187623478217404, -5.790488632116400858, -19.50000000000000355 ) ) ;
#27248=LINE ( 'NONE', #29738, #14877 ) ;
#27277=CARTESIAN_POINT ( 'NONE',  ( 26.80246859415415273, 7.028748154183637631, -1.499999999999999556 ) ) ;
#27279=FACE_OUTER_BOUND ( 'NONE', #20867, .T. ) ;
#27289=EDGE_CURVE ( 'NONE', #5438, #15872, #30527, .T. ) ;
#27306=ADVANCED_FACE ( 'NONE', ( #8095 ), #29765, .T. ) ;
#27317=VECTOR ( 'NONE', #13117, 1000.000000000000000 ) ;
#27360=AXIS2_PLACEMENT_3D ( 'NONE', #10566, #5885, #25060 ) ;
#27373=CARTESIAN_POINT ( 'NONE',  ( -13.22505861668333083, 42.10773672057167261, -19.50000000000000355 ) ) ;
#27377=ORIENTED_EDGE ( 'NONE', *, *, #19476, .T. ) ;
#27379=CARTESIAN_POINT ( 'NONE',  ( -10.11202017158235833, -41.14070756921188377, -1.500000000000000000 ) ) ;
#27381=DIRECTION ( 'NONE',  ( 0.5503133621338236470, 0.8349582046168341209, 0.000000000000000000 ) ) ;
#27384=CARTESIAN_POINT ( 'NONE',  ( 39.83602371822922095, -11.57901747687539640, -19.50000000000000355 ) ) ;
#27386=ORIENTED_EDGE ( 'NONE', *, *, #8502, .T. ) ;
#27387=AXIS2_PLACEMENT_3D ( 'NONE', #2553, #21559, #4885 ) ;
#27390=ORIENTED_EDGE ( 'NONE', *, *, #20240, .F. ) ;
#27395=B_SPLINE_CURVE_WITH_KNOTS ( 'NONE', 3,
 ( #12581, #7439, #16943, #23796, #3060, #17250, #26462, #26620, #28646, #253, #19587, #14451, #7745, #24266, #2599, #23954, #2756, #12118, #5247, #9926, #5092, #26776, #9620, #17093, #9766, #19278 ),
 .UNSPECIFIED., .F., .F.,
 ( 4, 2, 2, 2, 1, 2, 2, 2, 2, 2, 2, 1, 2, 4 ),
 ( 0.5002013267716731715, 0.5119551913427370371, 0.5237090559138010137, 0.5354629204848648794, 0.5413398527703968677, 0.5442783189131628063, 0.5472167850559288560, 0.5589706496269926106, 0.5707245141980563652, 0.5766014464835882425, 0.5824783787691202308, 0.5883553110546521081, 0.5912937771974180468, 0.5942322433401839854 ),
 .UNSPECIFIED. ) ;
#27399=CARTESIAN_POINT ( 'NONE',  ( -25.64627119138473432, -23.40052582045089480, -6.500000000000000888 ) ) ;
#27414=CARTESIAN_POINT ( 'NONE',  ( 40.89187623478217404, 5.790488632116406187, -19.50000000000000355 ) ) ;
#27473=EDGE_CURVE ( 'NONE', #21864, #24108, #7452, .T. ) ;
#27485=( NAMED_UNIT ( * ) PLANE_ANGLE_UNIT ( ) SI_UNIT ( $, .RADIAN. ) );
#27487=EDGE_CURVE ( 'NONE', #17387, #11174, #25062, .T. ) ;
#27508=CARTESIAN_POINT ( 'NONE',  ( -20.45518110071315832, -26.46109910111415431, -16.50001200000000168 ) ) ;
#27521=CARTESIAN_POINT ( 'NONE',  ( -25.19442432475474902, -35.44676296258422354, -19.50000000000000355 ) ) ;
#27526=CARTESIAN_POINT ( 'NONE',  ( 20.65888525914375862, -38.75220717792901581, -19.50000000000000355 ) ) ;
#27532=CARTESIAN_POINT ( 'NONE',  ( 10.64374042650142904, 42.96126232887663576, -19.50000000000000355 ) ) ;
#27559=ORIENTED_EDGE ( 'NONE', *, *, #6510, .T. ) ;
#27561=CARTESIAN_POINT ( 'NONE',  ( -39.83602371821029919, -11.57901747687044924, -19.50000000000000355 ) ) ;
#27589=DIRECTION ( 'NONE',  ( -0.000000000000000000, -0.000000000000000000, -1.000000000000000000 ) ) ;
#27605=LINE ( 'NONE', #6227, #18171 ) ;
#27620=CARTESIAN_POINT ( 'NONE',  ( -39.52380524536133777, -7.028748154183623420, -6.500000000000000888 ) ) ;
#27630=ORIENTED_EDGE ( 'NONE', *, *, #14536, .F. ) ;
#27633=DIRECTION ( 'NONE',  ( -0.000000000000000000, 0.000000000000000000, -1.000000000000000000 ) ) ;
#27640=DIRECTION ( 'NONE',  ( -1.000000000000000000, 0.000000000000000000, 0.000000000000000000 ) ) ;
#27644=CARTESIAN_POINT ( 'NONE',  ( 40.05104235265675783, 2.353288714454550234, -6.500000000000000888 ) ) ;
#27646=EDGE_LOOP ( 'NONE', ( #28784, #19207, #5331, #10240, #769, #4250, #5662, #11982 ) ) ;
#27651=CARTESIAN_POINT ( 'NONE',  ( -23.16753610420780873, -35.74416778164192010, -13.16661231005593713 ) ) ;
#27660=ORIENTED_EDGE ( 'NONE', *, *, #21127, .T. ) ;
#27661=CARTESIAN_POINT ( 'NONE',  ( 39.83602371821015709, 11.57901747687536265, -19.50000000000000355 ) ) ;
#27665=CARTESIAN_POINT ( 'NONE',  ( 10.11202017158463917, -41.14070756921186955, -1.500000000000000000 ) ) ;
#27666=CARTESIAN_POINT ( 'NONE',  ( -23.27838111883973227, 36.10018642694448943, -16.50000600000000262 ) ) ;
#27670=CARTESIAN_POINT ( 'NONE',  ( 10.11202017158463917, -41.14070756921186955, -1.500000000000000000 ) ) ;
#27674=CARTESIAN_POINT ( 'NONE',  ( 39.52380524533145945, -7.028748154382047808, -6.500000000000000888 ) ) ;
#27684=EDGE_LOOP ( 'NONE', ( #28449, #22339, #27377, #14857, #6752, #2699, #22375, #4443 ) ) ;
#27689=EDGE_CURVE ( 'NONE', #16328, #20004, #8637, .T. ) ;
#27690=DIRECTION ( 'NONE',  ( -0.000000000000000000, 0.000000000000000000, 1.000000000000000000 ) ) ;
#27706=ORIENTED_EDGE ( 'NONE', *, *, #17908, .T. ) ;
#27734=MECHANICAL_DESIGN_GEOMETRIC_PRESENTATION_REPRESENTATION('',(#24733),#14757);
#27739=VECTOR ( 'NONE', #6933, 1000.000000000000000 ) ;
#27765=CYLINDRICAL_SURFACE ( 'NONE', #6514, 1.447898107987198646 ) ;
#27766=ORIENTED_EDGE ( 'NONE', *, *, #12817, .F. ) ;
#27778=B_SPLINE_CURVE_WITH_KNOTS ( 'NONE', 3,
 ( #1754, #16106, #1907, #8634, #25626, #22815, #1466, #21069, #11270, #28114, #27965, #18145, #17998, #11433, #27508, #25150, #20920, #30296 ),
 .UNSPECIFIED., .F., .F.,
 ( 4, 2, 2, 2, 2, 2, 2, 2, 4 ),
 ( 0.000000000000000000, 0.1250000000000000000, 0.2500000000000000000, 0.3750000000000000000, 0.5000000000000000000, 0.6250000000000000000, 0.7500000000000000000, 0.8750000000000000000, 1.000000000000000000 ),
 .UNSPECIFIED. ) ;
#27779=AXIS2_PLACEMENT_3D ( 'NONE', #7051, #14535, #4557 ) ;
#27786=ADVANCED_FACE ( 'NONE', ( #18001 ), #30144, .F. ) ;
#27791=VECTOR ( 'NONE', #20192, 999.9999999999998863 ) ;
#27814=CARTESIAN_POINT ( 'NONE',  ( -23.00100564344168674, -35.20929534199333233, -8.166629675772911767 ) ) ;
#27835=DIRECTION ( 'NONE',  ( -1.000000000000000000, 0.000000000000000000, 0.000000000000000000 ) ) ;
#27840=CARTESIAN_POINT ( 'NONE',  ( -32.74775157610760346, -27.21557300919352329, -19.50000000000000355 ) ) ;
#27869=AXIS2_PLACEMENT_3D ( 'NONE', #20152, #29669, #22949 ) ;
#27870=VERTEX_POINT ( 'NONE', #23882 ) ;
#27872=CARTESIAN_POINT ( 'NONE',  ( 40.89187623478217404, -5.790488632116400858, -19.50000000000000355 ) ) ;
#27892=CARTESIAN_POINT ( 'NONE',  ( -39.87808514440047247, 7.028748154183623420, -14.83333104106490197 ) ) ;
#27898=EDGE_CURVE ( 'NONE', #13626, #2292, #9392, .T. ) ;
#27930=ORIENTED_EDGE ( 'NONE', *, *, #6331, .F. ) ;
#27940=ORIENTED_EDGE ( 'NONE', *, *, #13051, .T. ) ;
#27965=CARTESIAN_POINT ( 'NONE',  ( -21.14898501148481103, -24.45236287589831292, -16.50001200000000168 ) ) ;
#27974=CARTESIAN_POINT ( 'NONE',  ( 39.00000000000000000, -5.563236990218592304, -1.500000000000000000 ) ) ;
#28002=DIRECTION ( 'NONE',  ( -0.4539545692076746852, 0.8910248307962436165, 0.000000000000000000 ) ) ;
#28003=CARTESIAN_POINT ( 'NONE',  ( -24.03057240117691862, 26.57182937991349903, -6.500000000000000888 ) ) ;
#28011=CARTESIAN_POINT ( 'NONE',  ( -39.00000000000000000, -5.563236990218529243, -1.500000000000000000 ) ) ;
#28016=EDGE_CURVE ( 'NONE', #25162, #23566, #28569, .T. ) ;
#28026=EDGE_CURVE ( 'NONE', #29503, #26411, #7049, .T. ) ;
#28062=VERTEX_POINT ( 'NONE', #21856 ) ;
#28073=B_SPLINE_CURVE_WITH_KNOTS ( 'NONE', 3,
 ( #14018, #11222, #23376, #23210, #1864, #11389 ),
 .UNSPECIFIED., .F., .F.,
 ( 4, 2, 4 ),
 ( 0.001794032523745612293, 0.007046146517948603805, 0.01388807892444512623 ),
 .UNSPECIFIED. ) ;
#28078=EDGE_LOOP ( 'NONE', ( #26812, #7201 ) ) ;
#28088=B_SPLINE_SURFACE_WITH_KNOTS ( 'NONE', 1, 3, ( 
 ( #10059, #7884, #29088, #28939, #27061, #7730, #26602, #231, #9744, #19258, #7417, #26445, #17390, #5074, #12243, #29702, #27526, #20641, #15503, #3512, #25167, #15182, #10520, #8346, #25332, #15653, #25020, #13026, #22831, #1013, #12878, #24704, #1482, #22377, #3973, #22977, #18163, #6147, #20493, #8655, #29552, #17862 ),
 ( #10672, #22513, #27209, #1162, #13493, #3659, #3811, #10994, #5846, #13334, #20031, #8186, #11144, #22666, #15812, #30014, #15346, #30160, #27670, #8792, #18319, #6299, #1317, #27379, #5686, #24876, #5999, #3346, #13173, #10836, #20344, #29874, #8514, #14072, #11743, #30769, #23129, #23734, #6609, #23581, #6755, #16270 ) ),
 .UNSPECIFIED., .F., .T., .F.,
 ( 2, 2 ),
 ( 4, 2, 2, 2, 2, 2, 2, 2, 2, 2, 2, 2, 2, 2, 2, 2, 2, 2, 2, 2, 4 ),
 ( 0.000000000000000000, 1.000000000000000000 ),
 ( 0.000000000000000000, 0.1963495408493620697, 0.3926990816987241395, 0.7853981633974482790, 1.178097245096172418, 1.570796326794896558, 1.963495408493620697, 2.356194490192344837, 2.748893571891068976, 2.945243112740430824, 3.141592653589793116, 3.337942194439155408, 3.534291735288517255, 3.926990816987241395, 4.319689898685965090, 4.712388980384689674, 5.105088062083414258, 5.497787143782137953, 5.890486225480861648, 6.086835766330223940, 6.283185307179586232 ),
 .UNSPECIFIED. ) ;
#28108=CARTESIAN_POINT ( 'NONE',  ( -22.44164183933027701, 36.72099769060108088, -16.50000000000000000 ) ) ;
#28113=CARTESIAN_POINT ( 'NONE',  ( 2.168404344971008868E-16, 42.50000000000000711, -1.500000000000000000 ) ) ;
#28114=CARTESIAN_POINT ( 'NONE',  ( -21.37787209074186734, -24.17206580633116175, -16.50001200000000523 ) ) ;
#28134=ORIENTED_EDGE ( 'NONE', *, *, #4959, .F. ) ;
#28137=CARTESIAN_POINT ( 'NONE',  ( -2.552544031601109875, 42.50000000001772094, -1.500000000000000000 ) ) ;
#28139=ORIENTED_EDGE ( 'NONE', *, *, #7710, .T. ) ;
#28159=CARTESIAN_POINT ( 'NONE',  ( 32.82330813384650270, 22.94799032727486932, -1.500000000000000000 ) ) ;
#28198=ORIENTED_EDGE ( 'NONE', *, *, #1199, .F. ) ;
#28230=CARTESIAN_POINT ( 'NONE',  ( -25.64627119138473432, 23.40052582045089480, -16.50001200000000168 ) ) ;
#28234=EDGE_CURVE ( 'NONE', #12141, #7038, #1095, .T. ) ;
#28244=AXIS2_PLACEMENT_3D ( 'NONE', #28003, #15411, #3571 ) ;
#28246=EDGE_CURVE ( 'NONE', #3032, #21118, #11849, .T. ) ;
#28256=AXIS2_PLACEMENT_3D ( 'NONE', #29037, #19524, #334 ) ;
#28284=CARTESIAN_POINT ( 'NONE',  ( 37.98493438987956949, 11.12428508576150143, -1.500000000000000000 ) ) ;
#28328=CARTESIAN_POINT ( 'NONE',  ( 33.14492811172536335, 23.43596546612559806, -6.499905845448985531 ) ) ;
#28329=CARTESIAN_POINT ( 'NONE',  ( 10.11202017158399968, 41.14070756921128691, -1.500000000000000000 ) ) ;
#28352=DIRECTION ( 'NONE',  ( -0.000000000000000000, -0.000000000000000000, -1.000000000000000000 ) ) ;
#28354=B_SPLINE_SURFACE_WITH_KNOTS ( 'NONE', 3, 1, ( 
 ( #16848, #16531 ),
 ( #21508, #4991 ),
 ( #18885, #26049 ),
 ( #9669, #14503 ),
 ( #20991, #13848 ),
 ( #11196, #23030 ) ),
 .UNSPECIFIED., .F., .F., .F.,
 ( 4, 2, 4 ),
 ( 2, 2 ),
 ( 1.408367944312347353, 1.570796326794896558, 1.733224709277802811 ),
 ( 0.000000000000000000, 1.000000000000000000 ),
 .UNSPECIFIED. ) ;
#28380=ORIENTED_EDGE ( 'NONE', *, *, #27473, .F. ) ;
#28381=DIRECTION ( 'NONE',  ( 0.000000000000000000, 0.000000000000000000, -1.000000000000000000 ) ) ;
#28395=CARTESIAN_POINT ( 'NONE',  ( 39.52380524533145945, -7.028748154382047808, -11.49999999999999645 ) ) ;
#28396=CARTESIAN_POINT ( 'NONE',  ( 20.46975788395958418, -26.57181885929544407, -16.50000600000000262 ) ) ;
#28407=ORIENTED_EDGE ( 'NONE', *, *, #26912, .T. ) ;
#28426=CARTESIAN_POINT ( 'NONE',  ( -32.74775157610409337, 27.21557300919391054, -19.50000000000000355 ) ) ;
#28448=ADVANCED_FACE ( 'NONE', ( #16256 ), #22840, .T. ) ;
#28449=ORIENTED_EDGE ( 'NONE', *, *, #29903, .F. ) ;
#28453=ORIENTED_EDGE ( 'NONE', *, *, #12253, .T. ) ;
#28467=ORIENTED_EDGE ( 'NONE', *, *, #29177, .T. ) ;
#28468=VECTOR ( 'NONE', #9445, 1000.000000000000000 ) ;
#28471=FACE_OUTER_BOUND ( 'NONE', #17721, .T. ) ;
#28477=CARTESIAN_POINT ( 'NONE',  ( 31.18700685317242716, 26.11823559933198879, -1.500000000000000000 ) ) ;
#28497=CARTESIAN_POINT ( 'NONE',  ( -2.552544030762004645, -42.50000000000000000, -1.500000000000000000 ) ) ;
#28514=DIRECTION ( 'NONE',  ( 0.000000000000000000, 0.000000000000000000, 1.000000000000000000 ) ) ;
#28536=ORIENTED_EDGE ( 'NONE', *, *, #9979, .T. ) ;
#28541=CARTESIAN_POINT ( 'NONE',  ( 20.47140833542507821, 26.57182937991349903, -16.50000000000000000 ) ) ;
#28544=CARTESIAN_POINT ( 'NONE',  ( 39.52380524533145945, -7.028748154382047808, -6.500000000000000888 ) ) ;
#28545=CARTESIAN_POINT ( 'NONE',  ( -5.105024945673440229, 42.22604126506271882, -1.500000000000009992 ) ) ;
#28555=CARTESIAN_POINT ( 'NONE',  ( -24.03057240117690441, -26.57182937991348481, -1.500000000000001332 ) ) ;
#28563=CARTESIAN_POINT ( 'NONE',  ( -6.254902194515756797, 43.56090013333164279, -16.50000000000000000 ) ) ;
#28569=LINE ( 'NONE', #4705, #3861 ) ;
#28574=CARTESIAN_POINT ( 'NONE',  ( 34.07766914598172292, -21.40380666527112652, -1.500000000000000000 ) ) ;
#28581=CARTESIAN_POINT ( 'NONE',  ( 20.47140833542507821, 26.57182937991349903, -6.500000000000000888 ) ) ;
#28609=ORIENTED_EDGE ( 'NONE', *, *, #19661, .F. ) ;
#28610=CARTESIAN_POINT ( 'NONE',  ( 2.168404344971008868E-16, 42.50000000000000711, -1.500000000000000000 ) ) ;
#28611=CARTESIAN_POINT ( 'NONE',  ( 22.94541271837968566, 35.03073867843525591, -6.499999999999999112 ) ) ;
#28628=CARTESIAN_POINT ( 'NONE',  ( -10.11202017158466759, 41.14070756921185534, -1.500000000000000000 ) ) ;
#28639=ADVANCED_FACE ( 'NONE', ( #21190 ), #28354, .F. ) ;
#28646=CARTESIAN_POINT ( 'NONE',  ( 10.54213442295891667, 42.56985972894294434, -16.50000000000000711 ) ) ;
#28656=CARTESIAN_POINT ( 'NONE',  ( 0.000000000000000000, 0.000000000000000000, -16.50000000000000000 ) ) ;
#28658=EDGE_CURVE ( 'NONE', #26358, #12583, #30218, .T. ) ;
#28673=EDGE_CURVE ( 'NONE', #6009, #7019, #25943, .T. ) ;
#28697=ORIENTED_EDGE ( 'NONE', *, *, #187, .F. ) ;
#28699=CARTESIAN_POINT ( 'NONE',  ( 39.87350638640861433, 4.706224724276823146, -6.500000000000000888 ) ) ;
#28704=VECTOR ( 'NONE', #6177, 1000.000000000000000 ) ;
#28707=ORIENTED_EDGE ( 'NONE', *, *, #29217, .F. ) ;
#28727=DIRECTION ( 'NONE',  ( 0.000000000000000000, 0.000000000000000000, -1.000000000000000000 ) ) ;
#28733=CARTESIAN_POINT ( 'NONE',  ( 2.552544030762014415, -42.50000000000000000, -1.500000000000000000 ) ) ;
#28736=DIRECTION ( 'NONE',  ( -0.000000000000000000, -0.000000000000000000, -1.000000000000000000 ) ) ;
#28741=CARTESIAN_POINT ( 'NONE',  ( -37.98493438988128901, 11.12428508575241004, -1.500000000000000000 ) ) ;
#28746=ORIENTED_EDGE ( 'NONE', *, *, #23070, .T. ) ;
#28753=VERTEX_POINT ( 'NONE', #2131 ) ;
#28762=CARTESIAN_POINT ( 'NONE',  ( 31.31394823342230183, 25.51108937476774585, -1.500000000000003997 ) ) ;
#28784=ORIENTED_EDGE ( 'NONE', *, *, #26582, .F. ) ;
#28814=CIRCLE ( 'NONE', #17848, 3.559164065751841743 ) ;
#28837=DIRECTION ( 'NONE',  ( -0.000000000000000000, -1.000000000000000000, 0.000000000000000000 ) ) ;
#28860=CARTESIAN_POINT ( 'NONE',  ( -39.87808514257974224, -7.028748160228998287, -14.83333104093387611 ) ) ;
#28892=CARTESIAN_POINT ( 'NONE',  ( 10.64374042650304020, -42.96126232887725394, -19.50000000000000355 ) ) ;
#28899=CARTESIAN_POINT ( 'NONE',  ( -25.19442432475474902, -35.44676296258422354, -19.50000000000000355 ) ) ;
#28902=EDGE_CURVE ( 'NONE', #29503, #12213, #17709, .T. ) ;
#28905=CARTESIAN_POINT ( 'NONE',  ( 32.93066664481101924, -23.11087910253144528, -3.166603179814984959 ) ) ;
#28923=CARTESIAN_POINT ( 'NONE',  ( 19.82873939126788443, -38.47025822325555566, -16.50000000000000355 ) ) ;
#28934=B_SPLINE_CURVE_WITH_KNOTS ( 'NONE', 3,
 ( #28610, #9888, #30624, #11935, #18953, #26427, #21259, #26260, #28762, #16592 ),
 .UNSPECIFIED., .F., .F.,
 ( 4, 2, 2, 2, 4 ),
 ( 0.1275862231236772337, 0.1353932202260588469, 0.1432002173284404600, 0.1588142115332036863, 0.1673618661614010295 ),
 .UNSPECIFIED. ) ;
#28937=DIRECTION ( 'NONE',  ( -0.8910248307962436165, -0.4539545692076746852, 0.000000000000000000 ) ) ;
#28939=CARTESIAN_POINT ( 'NONE',  ( 10.64374042650142904, 42.96126232887663576, -19.50000000000000355 ) ) ;
#28947=ORIENTED_EDGE ( 'NONE', *, *, #8876, .F. ) ;
#28954=CARTESIAN_POINT ( 'NONE',  ( -10.11202017158235833, -41.14070756921188377, -1.500000000000000000 ) ) ;
#28964=EDGE_LOOP ( 'NONE', ( #13305, #12505 ) ) ;
#28979=CARTESIAN_POINT ( 'NONE',  ( 31.92585768969536630, 26.59981599185444878, -13.16665969302820471 ) ) ;
#29005=VECTOR ( 'NONE', #17684, 1000.000000000000000 ) ;
#29015=EDGE_LOOP ( 'NONE', ( #11811, #4035, #30691, #15226 ) ) ;
#29029=DIRECTION ( 'NONE',  ( 0.000000000000000000, 0.000000000000000000, -1.000000000000000000 ) ) ;
#29036=CARTESIAN_POINT ( 'NONE',  ( 40.89187623478217404, -5.790488632116400858, -19.50000000000000355 ) ) ;
#29037=CARTESIAN_POINT ( 'NONE',  ( 0.000000000000000000, 0.000000000000000000, -11.49999999999999645 ) ) ;
#29045=CARTESIAN_POINT ( 'NONE',  ( -20.65888525914364493, -38.75220717792906555, -19.50000000000000355 ) ) ;
#29046=EDGE_CURVE ( 'NONE', #8392, #16888, #25659, .T. ) ;
#29048=VECTOR ( 'NONE', #15640, 1000.000000000000114 ) ;
#29066=VECTOR ( 'NONE', #24764, 1000.000000000000114 ) ;
#29080=CARTESIAN_POINT ( 'NONE',  ( -5.729465025513086419E-13, 44.07656359094158915, -16.50000000000000000 ) ) ;
#29088=CARTESIAN_POINT ( 'NONE',  ( 5.374868878255610660, 44.10336124695606230, -19.50000000000000355 ) ) ;
#29141=EDGE_LOOP ( 'NONE', ( #28198, #28380, #6878, #16003, #21226, #27390, #14658, #27559 ) ) ;
#29158=DIRECTION ( 'NONE',  ( -1.000000000000000000, 0.000000000000000000, 0.000000000000000000 ) ) ;
#29174=AXIS2_PLACEMENT_3D ( 'NONE', #4476, #26134, #7429 ) ;
#29177=EDGE_CURVE ( 'NONE', #14731, #11716, #14777, .T. ) ;
#29184=DIRECTION ( 'NONE',  ( -1.000000000000000000, 0.000000000000000000, 0.000000000000000000 ) ) ;
#29186=EDGE_CURVE ( 'NONE', #18557, #13268, #16365, .T. ) ;
#29188=CARTESIAN_POINT ( 'NONE',  ( -5.105024945673440229, 42.22604126506271172, -1.500000000000000000 ) ) ;
#29194=DIRECTION ( 'NONE',  ( 0.5503133621338236470, -0.8349582046168341209, 0.000000000000000000 ) ) ;
#29196=CARTESIAN_POINT ( 'NONE',  ( 5.105024945673418912, -42.22604126506271882, -1.500000000000000000 ) ) ;
#29203=AXIS2_PLACEMENT_3D ( 'NONE', #3829, #27690, #11468 ) ;
#29217=EDGE_CURVE ( 'NONE', #13626, #20319, #30301, .T. ) ;
#29218=CARTESIAN_POINT ( 'NONE',  ( -25.23756106473024019, 11.43858098102958287, -11.49999999999999645 ) ) ;
#29258=ORIENTED_EDGE ( 'NONE', *, *, #28658, .F. ) ;
#29259=DIRECTION ( 'NONE',  ( -1.000000000000000000, 0.000000000000000000, -0.000000000000000000 ) ) ;
#29282=VERTEX_POINT ( 'NONE', #24534 ) ;
#29297=EDGE_CURVE ( 'NONE', #544, #13676, #19868, .T. ) ;
#29338=CARTESIAN_POINT ( 'NONE',  ( 20.71335220384823117, 27.86167394782616213, -16.50000000000000000 ) ) ;
#29351=ORIENTED_EDGE ( 'NONE', *, *, #11073, .T. ) ;
#29363=CARTESIAN_POINT ( 'NONE',  ( -12.56641067637617759, -40.32935944494947478, -1.500000000000000000 ) ) ;
#29372=VERTEX_POINT ( 'NONE', #3328 ) ;
#29406=EDGE_LOOP ( 'NONE', ( #13427, #10558, #20851, #6163 ) ) ;
#29411=CARTESIAN_POINT ( 'NONE',  ( -20.71335220384823117, -27.86167394782616213, -6.500000000000000888 ) ) ;
#29435=ADVANCED_FACE ( 'NONE', ( #9690, #2366 ), #7520, .T. ) ;
#29452=CARTESIAN_POINT ( 'NONE',  ( 40.48994520213110349, 2.927201920381877542, -16.49999999999999645 ) ) ;
#29503=VERTEX_POINT ( 'NONE', #5641 ) ;
#29517=CARTESIAN_POINT ( 'NONE',  ( -22.58267429318970443, -26.57182937991348481, -6.499999999999999112 ) ) ;
#29547=CARTESIAN_POINT ( 'NONE',  ( 25.19442432474404470, 35.44676296256560022, -19.50000000000000355 ) ) ;
#29549=ORIENTED_EDGE ( 'NONE', *, *, #187, .T. ) ;
#29552=CARTESIAN_POINT ( 'NONE',  ( -2.687479363073305372, 44.39187623477332068, -19.50000000000000355 ) ) ;
#29589=CARTESIAN_POINT ( 'NONE',  ( -25.19442432475474902, -35.44676296258422354, -19.50000000000000355 ) ) ;
#29622=LINE ( 'NONE', #17764, #29996 ) ;
#29623=ORIENTED_EDGE ( 'NONE', *, *, #27112, .F. ) ;
#29635=ORIENTED_EDGE ( 'NONE', *, *, #4058, .F. ) ;
#29641=ORIENTED_EDGE ( 'NONE', *, *, #13909, .T. ) ;
#29644=EDGE_CURVE ( 'NONE', #23566, #28062, #7093, .T. ) ;
#29658=CARTESIAN_POINT ( 'NONE',  ( 24.03057240117691862, 26.57182937991349903, -6.500000000000000888 ) ) ;
#29664=( LENGTH_UNIT ( ) NAMED_UNIT ( * ) SI_UNIT ( .MILLI., .METRE. ) );
#29669=DIRECTION ( 'NONE',  ( -0.000000000000000000, -0.000000000000000000, -1.000000000000000000 ) ) ;
#29672=CARTESIAN_POINT ( 'NONE',  ( 0.000000000000000000, 0.000000000000000000, -6.500000000000000888 ) ) ;
#29684=CARTESIAN_POINT ( 'NONE',  ( -20.50469103882543109, 27.17502484134975305, -16.50001200000000523 ) ) ;
#29689=DIRECTION ( 'NONE',  ( -0.2972711322815274615, 0.9547931052914336858, 0.000000000000000000 ) ) ;
#29694=PLANE ( 'NONE',  #22739 ) ;
#29695=CARTESIAN_POINT ( 'NONE',  ( 34.07766914600081520, 21.40380666527109810, -1.500000000000000000 ) ) ;
#29697=CARTESIAN_POINT ( 'NONE',  ( -23.11204206675364503, 35.56592873118525944, -11.49994521161821481 ) ) ;
#29702=CARTESIAN_POINT ( 'NONE',  ( 25.19442432473618254, -35.44676296258426618, -19.50000000000000355 ) ) ;
#29708=CARTESIAN_POINT ( 'NONE',  ( 25.19442432473618254, -35.44676296258426618, -19.50000000000000355 ) ) ;
#29714=EDGE_LOOP ( 'NONE', ( #28697, #2580, #7248, #15179 ) ) ;
#29738=CARTESIAN_POINT ( 'NONE',  ( 0.000000000000000000, 7.028748154183637631, -16.50000000000000000 ) ) ;
#29751=CARTESIAN_POINT ( 'NONE',  ( -4.433228896135648966, -43.81350511682552451, -16.50000000000000000 ) ) ;
#29765=PLANE ( 'NONE',  #12605 ) ;
#29771=CYLINDRICAL_SURFACE ( 'NONE', #11775, 27.70876437800068359 ) ;
#29778=CARTESIAN_POINT ( 'NONE',  ( 39.87808514434166085, -7.028748154387577607, -14.83333104074398356 ) ) ;
#29792=VECTOR ( 'NONE', #4586, 1000.000000000000114 ) ;
#29810=ORIENTED_EDGE ( 'NONE', *, *, #21390, .T. ) ;
#29868=CARTESIAN_POINT ( 'NONE',  ( 10.64374042650142904, 42.96126232887663576, -19.50000000000000355 ) ) ;
#29871=EDGE_LOOP ( 'NONE', ( #29952, #29623, #601, #28947 ) ) ;
#29874=CARTESIAN_POINT ( 'NONE',  ( -39.00000000000000000, 5.563236990218665134, -1.500000000000000000 ) ) ;
#29876=LINE ( 'NONE', #8516, #9591 ) ;
#29879=CARTESIAN_POINT ( 'NONE',  ( 40.89187623478217404, 5.790488632116406187, -19.50000000000000355 ) ) ;
#29895=CARTESIAN_POINT ( 'NONE',  ( -7.500000000000000000, 0.000000000000000000, -1.500000000000001332 ) ) ;
#29903=EDGE_CURVE ( 'NONE', #24108, #20004, #11796, .T. ) ;
#29910=FACE_OUTER_BOUND ( 'NONE', #4091, .T. ) ;
#29912=EDGE_LOOP ( 'NONE', ( #15342, #14314, #2902, #14937 ) ) ;
#29952=ORIENTED_EDGE ( 'NONE', *, *, #10269, .F. ) ;
#29965=ORIENTED_EDGE ( 'NONE', *, *, #24280, .T. ) ;
#29981=DIRECTION ( 'NONE',  ( 1.000000000000000000, 0.000000000000000000, 0.000000000000000000 ) ) ;
#29982=EDGE_CURVE ( 'NONE', #16098, #4045, #20804, .T. ) ;
#29996=VECTOR ( 'NONE', #28736, 1000.000000000000000 ) ;
#30002=EDGE_CURVE ( 'NONE', #2231, #15872, #2442, .T. ) ;
#30003=ORIENTED_EDGE ( 'NONE', *, *, #11651, .T. ) ;
#30005=CARTESIAN_POINT ( 'NONE',  ( 35.76344986165623396, 22.29344514668041199, -19.50000000000000355 ) ) ;
#30010=CARTESIAN_POINT ( 'NONE',  ( -5.374868878256215510, -44.10336124695545124, -19.50000000000000355 ) ) ;
#30014=CARTESIAN_POINT ( 'NONE',  ( 23.96732207938043402, -33.98584080152387088, -1.500000000000000000 ) ) ;
#30021=CARTESIAN_POINT ( 'NONE',  ( 0.000000000000000000, 44.39187623478217404, -19.50000000000000355 ) ) ;
#30045=ORIENTED_EDGE ( 'NONE', *, *, #23145, .T. ) ;
#30047=CARTESIAN_POINT ( 'NONE',  ( 35.76344986163714168, -22.29344514668044752, -19.50000000000000355 ) ) ;
#30062=ORIENTED_EDGE ( 'NONE', *, *, #6175, .T. ) ;
#30126=ORIENTED_EDGE ( 'NONE', *, *, #15674, .T. ) ;
#30130=ORIENTED_EDGE ( 'NONE', *, *, #20072, .F. ) ;
#30144=CYLINDRICAL_SURFACE ( 'NONE', #9328, 1.447898107987198646 ) ;
#30155=CARTESIAN_POINT ( 'NONE',  ( 34.07766914598172292, -21.40380666527112652, -1.500000000000000000 ) ) ;
#30156=CARTESIAN_POINT ( 'NONE',  ( 32.81350286003733885, 0.000000000000000000, -6.500000000000000888 ) ) ;
#30160=CARTESIAN_POINT ( 'NONE',  ( 12.56641067637628240, -40.32935944494942504, -1.500000000000000000 ) ) ;
#30164=CARTESIAN_POINT ( 'NONE',  ( -25.23756106473024374, 11.43858098102958110, -16.50000000000000000 ) ) ;
#30197=CARTESIAN_POINT ( 'NONE',  ( -5.374868878256215510, -44.10336124695545124, -19.50000000000000355 ) ) ;
#30218=LINE ( 'NONE', #14130, #7871 ) ;
#30220=DIRECTION ( 'NONE',  ( 0.000000000000000000, 0.000000000000000000, -1.000000000000000000 ) ) ;
#30223=CARTESIAN_POINT ( 'NONE',  ( -39.52380524536136619, -7.028748154183644736, -11.49999999999999645 ) ) ;
#30253=LINE ( 'NONE', #3447, #22540 ) ;
#30296=CARTESIAN_POINT ( 'NONE',  ( -20.71335220384823117, -27.86167394782616213, -16.50000000000000000 ) ) ;
#30301=CIRCLE ( 'NONE', #16855, 27.70876437800068359 ) ;
#30308=CARTESIAN_POINT ( 'NONE',  ( -31.18700685316100163, -26.11823559932341610, -1.500000000000000000 ) ) ;
#30319=CARTESIAN_POINT ( 'NONE',  ( -23.96732207939035675, 33.98584080153585774, -1.500000000000000000 ) ) ;
#30328=VERTEX_POINT ( 'NONE', #22474 ) ;
#30329=CARTESIAN_POINT ( 'NONE',  ( -31.76816150360384228, 26.51947378168403091, -11.49999299997503499 ) ) ;
#30342=CARTESIAN_POINT ( 'NONE',  ( 32.24119435725080507, -26.76047165977712794, -16.50000600000000262 ) ) ;
#30343=LINE ( 'NONE', #21113, #20983 ) ;
#30354=CARTESIAN_POINT ( 'NONE',  ( 34.07766914598172292, -21.40380666527112652, -1.500000000000000000 ) ) ;
#30361=CYLINDRICAL_SURFACE ( 'NONE', #13183, 3.559164065751841743 ) ;
#30362=ADVANCED_FACE ( 'NONE', ( #7685 ), #17183, .F. ) ;
#30377=VERTEX_POINT ( 'NONE', #22172 ) ;
#30378=DIRECTION ( 'NONE',  ( -1.000000000000000000, 0.000000000000000000, 0.000000000000000000 ) ) ;
#30380=CARTESIAN_POINT ( 'NONE',  ( 14.28398042828922421, -41.31607170670246632, -16.50000000000000000 ) ) ;
#30411=LINE ( 'NONE', #18564, #18635 ) ;
#30464=CARTESIAN_POINT ( 'NONE',  ( -12.56641067637752229, 40.32935944495016400, -1.500000000000000000 ) ) ;
#30490=CARTESIAN_POINT ( 'NONE',  ( 19.64114023396309960, -37.13592150529014191, -1.500000000000000000 ) ) ;
#30494=CARTESIAN_POINT ( 'NONE',  ( 31.18700685317022803, -26.11823559933272421, -1.500000000000000000 ) ) ;
#30502=CARTESIAN_POINT ( 'NONE',  ( -33.03787111873038640, -23.27353416640910311, -4.833238796522825176 ) ) ;
#30517=EDGE_CURVE ( 'NONE', #23101, #2292, #14184, .T. ) ;
#30527=B_SPLINE_CURVE_WITH_KNOTS ( 'NONE', 3,
 ( #12307, #5444, #15091, #21809, #285, #911, #14481 ),
 .UNSPECIFIED., .F., .F.,
 ( 4, 3, 4 ),
 ( 0.000000000000000000, 0.005028111721449823532, 0.01005622344637598607 ),
 .UNSPECIFIED. ) ;
#30530=EDGE_LOOP ( 'NONE', ( #1912, #26259, #24054, #16610 ) ) ;
#30540=FACE_OUTER_BOUND ( 'NONE', #29912, .T. ) ;
#30561=EDGE_CURVE ( 'NONE', #4972, #6254, #28814, .T. ) ;
#30568=CARTESIAN_POINT ( 'NONE',  ( 39.87350638640253919, -4.706224724400470016, -6.500000000000000888 ) ) ;
#30586=CARTESIAN_POINT ( 'NONE',  ( -3.661196020523152406, 43.90033885078650400, -16.50000000000000000 ) ) ;
#30589=LINE ( 'NONE', #9229, #6314 ) ;
#30602=CARTESIAN_POINT ( 'NONE',  ( -37.98493438988128901, 11.12428508575241004, -1.500000000000000000 ) ) ;
#30603=CARTESIAN_POINT ( 'NONE',  ( 2.687479363073301819, 44.39187623479102740, -19.50000000000000355 ) ) ;
#30624=CARTESIAN_POINT ( 'NONE',  ( 5.105024945674004222, 42.22604126506330857, -1.500000000000003997 ) ) ;
#30627=CARTESIAN_POINT ( 'NONE',  ( -25.23756106473024730, -11.43858098102957577, -1.500000000000000000 ) ) ;
#30635=CARTESIAN_POINT ( 'NONE',  ( 39.70095622559083637, -7.028748154384818925, -13.16666434783602924 ) ) ;
#30640=CARTESIAN_POINT ( 'NONE',  ( 33.03787111873281646, 23.27353416641277661, -4.833238796522779879 ) ) ;
#30641=CARTESIAN_POINT ( 'NONE',  ( 37.98493438989863336, -11.12428508576153341, -1.500000000000000000 ) ) ;
#30649=CARTESIAN_POINT ( 'NONE',  ( -33.25198511595942819, -23.59839678289454667, -8.166573069426220854 ) ) ;
#30656=VECTOR ( 'NONE', #11401, 1000.000000000000227 ) ;
#30681=CIRCLE ( 'NONE', #2823, 1.447898107987198646 ) ;
#30691=ORIENTED_EDGE ( 'NONE', *, *, #17028, .F. ) ;
#30725=VERTEX_POINT ( 'NONE', #3580 ) ;
#30755=CARTESIAN_POINT ( 'NONE',  ( 32.74775157612609178, -27.21557300919356948, -19.50000000000000355 ) ) ;
#30766=AXIS2_PLACEMENT_3D ( 'NONE', #1655, #8211, #17889 ) ;
#30768=DIRECTION ( 'NONE',  ( -0.000000000000000000, -0.000000000000000000, 1.000000000000000000 ) ) ;
#30769=CARTESIAN_POINT ( 'NONE',  ( -23.96732207939035675, 33.98584080153585774, -1.500000000000000000 ) ) ;
#30794=CIRCLE ( 'NONE', #924, 1.447898107987198646 ) ;
#30803=CARTESIAN_POINT ( 'NONE',  ( 33.35889462893408819, 23.76060431982160281, -9.833271596736157250 ) ) ;
#30804=CARTESIAN_POINT ( 'NONE',  ( 23.96732207937828463, 33.98584080152456011, -1.500000000000000000 ) ) ;
#30817=CARTESIAN_POINT ( 'NONE',  ( -11.29700601561300743, -42.33790872007643458, -16.50000000000000355 ) ) ;
#30831=FACE_OUTER_BOUND ( 'NONE', #14747, .T. ) ;
#30855=FACE_OUTER_BOUND ( 'NONE', #21240, .T. ) ;
#30887=COLOUR_RGB('Sky Blue',0.24,0.69,0.87);
#30888=FILL_AREA_STYLE_COLOUR('',#30887);
#30889=FILL_AREA_STYLE('',(#30888));
#30890=SURFACE_STYLE_FILL_AREA(#30889);
#30891=SURFACE_SIDE_STYLE('',(#30890));
#30892=SURFACE_STYLE_USAGE(.BOTH.,#30891);
#30893=PRESENTATION_STYLE_ASSIGNMENT((#30892));
ENDSEC;
END-ISO-10303-21;
